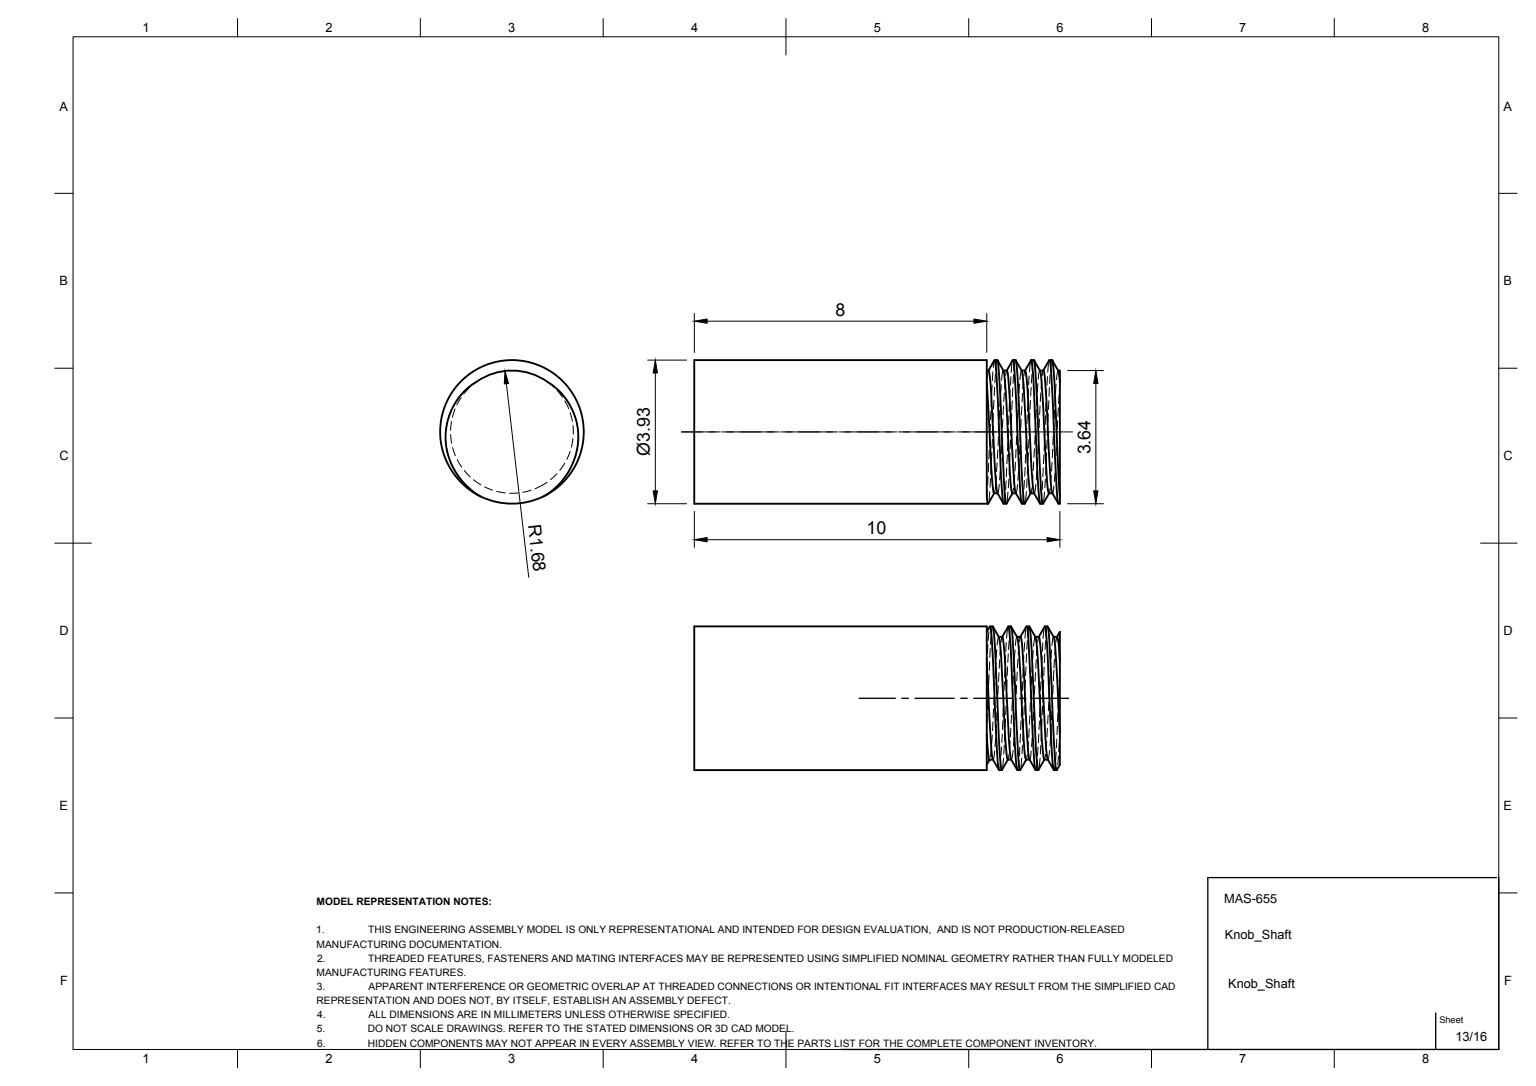
ISO-10303-21;
HEADER;
FILE_DESCRIPTION((''),'2;1');
FILE_NAME('Knob_Shaft.step','2026-10-09T11:34:15-07:00',(''),(''),'','','');
FILE_SCHEMA (('AUTOMOTIVE_DESIGN { 1 0 10303 214 3 1 1 }'));
ENDSEC;
DATA;
#10=MECHANICAL_DESIGN_GEOMETRIC_PRESENTATION_REPRESENTATION('',(#645),#117170);
#603=SHAPE_REPRESENTATION_RELATIONSHIP('SRR','None',#117258,#624) ;
#624=ADVANCED_BREP_SHAPE_REPRESENTATION('',(#666),#117166) ;
#645=STYLED_ITEM('',(#117355),#666) ;
#666=MANIFOLD_SOLID_BREP('Body1',#49074) ;
#761=FACE_BOUND('',#16411,.T.) ;
#1329=B_SPLINE_CURVE_WITH_KNOTS('',3,(#98755,#98756,#98757,#98758,#98759,
#98760,#98761,#98762,#98763,#98764,#98765,#98766,#98767,#98768,#98769,#98770,
#98771,#98772,#98773,#98774,#98775,#98776,#98777,#98778,#98779,#98780,#98781,
#98782,#98783,#98784,#98785,#98786,#98787,#98788,#98789,#98790,#98791,#98792,
#98793,#98794,#98795,#98796,#98797,#98798,#98799,#98800,#98801,#98802,#98803,
#98804,#98805,#98806,#98807,#98808,#98809,#98810,#98811,#98812,#98813,#98814,
#98815,#98816,#98817,#98818,#98819,#98820,#98821,#98822,#98823,#98824,#98825,
#98826,#98827,#98828,#98829,#98830,#98831,#98832,#98833,#98834),
 .UNSPECIFIED.,.F.,.F.,(4,2,2,2,2,2,2,2,2,2,2,2,2,2,2,2,2,2,2,2,2,2,2,2,
2,2,2,2,2,2,2,2,2,2,2,2,2,2,2,4),(-0.552597174673262,-0.552087978909823,
-0.543418802839412,-0.530986321926872,-0.515688074017889,-0.48901852632236,
-0.475795340291992,-0.469803806354904,-0.464827465085121,-0.456763485566357,
-0.446125790999932,-0.412222627640349,-0.396458552376544,-0.387367130961374,
-0.378547259036367,-0.364712615477276,-0.330180734182639,-0.312888098213682,
-0.306688567552087,-0.301731961915121,-0.294013236156573,-0.284057413245719,
-0.255750077060834,-0.235801635191627,-0.226007051069487,-0.217361674208648,
-0.205388809034252,-0.190982053575729,-0.163245460668606,-0.148987082829673,
-0.143002701370855,-0.137919038363949,-0.129466900901552,-0.118084610051148,
-0.0761832714464343,-0.0655381220499832,-0.0569431610964917,-0.0461350849955365,
-0.0209625497341524,-0.00261038353153479),.UNSPECIFIED.) ;
#1330=B_SPLINE_CURVE_WITH_KNOTS('',3,(#98837,#98838,#98839,#98840,#98841,
#98842,#98843,#98844,#98845,#98846,#98847,#98848,#98849,#98850,#98851,#98852,
#98853,#98854,#98855,#98856,#98857,#98858,#98859,#98860,#98861,#98862,#98863,
#98864,#98865,#98866,#98867,#98868,#98869,#98870,#98871,#98872,#98873,#98874,
#98875,#98876,#98877,#98878,#98879,#98880,#98881,#98882,#98883,#98884,#98885,
#98886),.UNSPECIFIED.,.F.,.F.,(4,2,2,2,2,2,2,2,2,2,2,2,2,2,2,2,2,2,2,2,
2,2,2,2,4),(-1.74405659608,-1.74024862573011,-1.7354490695973,-1.69761675650509,
-1.68391129329674,-1.67222759893424,-1.66298762114359,-1.6513941256668,
-1.6159137516185,-1.59065618245596,-1.58351862500578,-1.57860240737983,
-1.57213220939518,-1.537477246215,-1.51410228040979,-1.50437755876619,-1.49602419307963,
-1.48490892270242,-1.45580246644061,-1.43518707323026,-1.42657793655706,
-1.41966295247194,-1.41491213816115,-1.40875298679861,-1.40019423751868),
 .UNSPECIFIED.) ;
#1331=B_SPLINE_CURVE_WITH_KNOTS('',3,(#98891,#98892,#98893,#98894,#98895,
#98896,#98897,#98898,#98899,#98900,#98901,#98902,#98903,#98904,#98905,#98906,
#98907,#98908,#98909,#98910,#98911,#98912,#98913,#98914,#98915,#98916,#98917,
#98918,#98919,#98920,#98921,#98922,#98923,#98924,#98925,#98926,#98927,#98928,
#98929,#98930,#98931,#98932,#98933,#98934,#98935,#98936,#98937,#98938,#98939,
#98940,#98941,#98942,#98943,#98944,#98945,#98946,#98947,#98948,#98949,#98950,
#98951,#98952,#98953,#98954,#98955,#98956,#98957,#98958,#98959,#98960,#98961,
#98962,#98963,#98964,#98965,#98966,#98967,#98968,#98969,#98970,#98971,#98972,
#98973,#98974,#98975,#98976,#98977,#98978,#98979,#98980,#98981,#98982,#98983,
#98984,#98985,#98986,#98987,#98988,#98989,#98990,#98991,#98992,#98993,#98994,
#98995,#98996,#98997,#98998,#98999,#99000,#99001,#99002,#99003,#99004,#99005,
#99006,#99007,#99008,#99009,#99010,#99011,#99012,#99013,#99014,#99015,#99016,
#99017,#99018,#99019,#99020,#99021,#99022,#99023,#99024,#99025,#99026,#99027,
#99028,#99029,#99030,#99031,#99032),.UNSPECIFIED.,.F.,.F.,(4,2,2,2,2,2,
2,2,2,2,2,2,2,2,2,2,2,2,2,2,2,2,2,2,2,2,2,2,2,2,2,2,2,2,2,2,2,2,2,2,2,2,
2,2,2,2,2,2,2,2,2,2,2,2,2,2,2,2,2,2,2,2,2,2,2,2,2,2,2,2,4),(-1.60817871985196,
-1.60188697181691,-1.56617428509184,-1.54984087223545,-1.53688654692764,
-1.52815941900595,-1.51880035364366,-1.50119252756857,-1.46500106568252,
-1.45686511127176,-1.45016915517214,-1.4452730535428,-1.43827422610191,
-1.410720873795,-1.38068642007219,-1.37024130049903,-1.36171438017231,-1.35090239215872,
-1.31818186378263,-1.29333652168782,-1.28676822558853,-1.28186617089387,
-1.27471523608405,-1.25426210693583,-1.22954377855377,-1.21768281934354,
-1.20715919419871,-1.19863292932375,-1.18790517373592,-1.15426873354839,
-1.13057394980088,-1.12379973616585,-1.11890417570126,-1.11198677312076,
-1.08351739597117,-1.05355856892254,-1.04333843073385,-1.03479834540627,
-1.0238910563505,-0.996287106129177,-0.976227453852334,-0.964288354181759,
-0.958706935650863,-0.953530612564683,-0.944174280916242,-0.930866568317175,
-0.891101252113233,-0.880607430471217,-0.872083906506385,-0.861333132529412,
-0.836212201841313,-0.803368395572518,-0.796967637358088,-0.792061871113417,
-0.784846056910506,-0.775799271108273,-0.753119298036319,-0.728813193822705,
-0.717960451683399,-0.709427961265852,-0.69900655346212,-0.687320352856108,
-0.663461993928104,-0.641640554378349,-0.634492327931047,-0.62958458215972,
-0.622992165537731,-0.615037058215324,-0.580754809747541,-0.561631838713906,
-0.552597174673262),.UNSPECIFIED.) ;
#1332=B_SPLINE_CURVE_WITH_KNOTS('',3,(#99033,#99034,#99035,#99036,#99037,
#99038,#99039,#99040,#99041,#99042,#99043,#99044,#99045,#99046,#99047,#99048,
#99049,#99050,#99051,#99052,#99053,#99054,#99055,#99056,#99057,#99058,#99059,
#99060,#99061,#99062,#99063,#99064,#99065,#99066,#99067,#99068,#99069,#99070,
#99071,#99072,#99073,#99074,#99075,#99076,#99077,#99078,#99079,#99080,#99081,
#99082,#99083,#99084,#99085,#99086,#99087,#99088,#99089,#99090,#99091,#99092,
#99093,#99094,#99095,#99096,#99097,#99098,#99099,#99100,#99101,#99102,#99103,
#99104,#99105,#99106,#99107,#99108,#99109,#99110,#99111,#99112,#99113,#99114,
#99115,#99116,#99117,#99118,#99119,#99120,#99121,#99122,#99123,#99124,#99125,
#99126,#99127,#99128,#99129,#99130,#99131,#99132,#99133,#99134,#99135,#99136,
#99137,#99138,#99139,#99140,#99141,#99142,#99143,#99144,#99145,#99146,#99147,
#99148,#99149,#99150,#99151,#99152,#99153,#99154,#99155,#99156,#99157,#99158,
#99159,#99160,#99161,#99162,#99163,#99164,#99165,#99166,#99167,#99168,#99169,
#99170,#99171,#99172,#99173,#99174),.UNSPECIFIED.,.F.,.F.,(4,2,2,2,2,2,
2,2,2,2,2,2,2,2,2,2,2,2,2,2,2,2,2,2,2,2,2,2,2,2,2,2,2,2,2,2,2,2,2,2,2,2,
2,2,2,2,2,2,2,2,2,2,2,2,2,2,2,2,2,2,2,2,2,2,2,2,2,2,2,2,4),(-1.40019423751868,
-1.39059856461891,-1.35667598468847,-1.34290959713784,-1.33402342554946,
-1.32475733166678,-1.30815172066439,-1.27149851334997,-1.26331601166393,
-1.25658126033718,-1.25163113413534,-1.24446124954234,-1.22317299546722,
-1.19893660798004,-1.18715522406132,-1.17666499379619,-1.16809990650696,
-1.1572276585662,-1.12501053474387,-1.10009161766894,-1.09338700792244,
-1.08848701787225,-1.08148107106248,-1.05412084897453,-1.02341461347077,
-1.01315335487947,-1.00465968991157,-0.993932385879927,-0.961647123834745,
-0.936270329728169,-0.929746618015904,-0.92485572071812,-0.917705462014288,
-0.896911887819304,-0.872394270882754,-0.856049781705572,-0.846849723712218,
-0.838025885909813,-0.824390338136546,-0.790915249737361,-0.772823406769396,
-0.766455259867575,-0.761540972127907,-0.754256062725515,-0.745085604668567,
-0.721717226155916,-0.698227847610382,-0.687432671047302,-0.678903412564833,
-0.668436939858761,-0.637290397758027,-0.610963216220392,-0.603901842352647,
-0.599004302864263,-0.592366007013439,-0.56867953784493,-0.534621186939995,
-0.523939302554265,-0.515418012823645,-0.504864049701461,-0.492948449919942,
-0.467963543295212,-0.447868495117718,-0.440716118091854,-0.435815634952121,
-0.429254383948027,-0.40396129016647,-0.371801441673548,-0.360942278777566,
-0.35241374076114,-0.344414753026734),.UNSPECIFIED.) ;
#1333=B_SPLINE_CURVE_WITH_KNOTS('',3,(#99180,#99181,#99182,#99183,#99184,
#99185,#99186,#99187),.UNSPECIFIED.,.F.,.F.,(4,1,1,1,1,4),(21.9911559755827,
22.8773584072894,23.848998189505,24.8206379717207,25.7922777539364,26.2282473494963),
 .UNSPECIFIED.) ;
#1334=B_SPLINE_CURVE_WITH_KNOTS('',3,(#99188,#99189,#99190,#99191,#99192,
#99193,#99194,#99195,#99196,#99197,#99198,#99199,#99200,#99201,#99202,#99203,
#99204,#99205,#99206,#99207,#99208,#99209,#99210,#99211,#99212,#99213,#99214,
#99215,#99216,#99217,#99218,#99219,#99220,#99221,#99222,#99223,#99224,#99225,
#99226,#99227,#99228,#99229,#99230,#99231,#99232,#99233,#99234,#99235,#99236,
#99237),.UNSPECIFIED.,.F.,.F.,(4,2,2,2,2,2,2,2,2,2,2,2,2,2,2,2,2,2,2,2,
2,2,2,2,4),(-1.95186686044663,-1.9451727728085,-1.93967548024574,-1.93493962460603,
-1.92792572995927,-1.90152501587077,-1.87059969230919,-1.86007646778741,
-1.85155154543861,-1.84082680150995,-1.80717942800767,-1.78322121868641,
-1.77657104095611,-1.77167346878357,-1.76462252246752,-1.73795912356653,
-1.70712279558588,-1.69668728374485,-1.68816018090868,-1.67733734324366,
-1.64474656626435,-1.6204670242381,-1.61360536890348,-1.60871139946509,
-1.60817871985196),.UNSPECIFIED.) ;
#1335=B_SPLINE_CURVE_WITH_KNOTS('',3,(#99239,#99240,#99241,#99242,#99243,
#99244,#99245,#99246,#99247,#99248,#99249,#99250,#99251,#99252,#99253,#99254,
#99255,#99256,#99257,#99258,#99259,#99260,#99261,#99262,#99263,#99264,#99265,
#99266,#99267,#99268,#99269,#99270,#99271,#99272,#99273,#99274,#99275,#99276,
#99277,#99278,#99279,#99280,#99281,#99282,#99283,#99284,#99285,#99286,#99287,
#99288),.UNSPECIFIED.,.F.,.F.,(4,2,2,2,2,2,2,2,2,2,2,2,2,2,2,2,2,2,2,2,
2,2,2,2,4),(-0.344414753026734,-0.342008927015211,-0.330348848139387,-0.306608071890107,
-0.284590171653946,-0.277445774946498,-0.272544248501529,-0.265971783203178,
-0.240098440585068,-0.20869911101062,-0.197899738456524,-0.189367850672706,
-0.179070471921566,-0.14943964187475,-0.120798932996502,-0.113894953777187,
-0.109001470737898,-0.102221682855731,-0.0939417781600824,-0.0750956593381936,
-0.0453269004351953,-0.0345663159816099,-0.0260362888104047,-0.0179340362145887,
-0.000450587274275642),.UNSPECIFIED.) ;
#1336=B_SPLINE_CURVE_WITH_KNOTS('',3,(#99289,#99290,#99291,#99292,#99293,
#99294,#99295,#99296,#99297),.UNSPECIFIED.,.F.,.F.,(4,1,1,1,1,1,4),(21.991153076628,
22.3032518321271,23.2748916143428,24.2465313965585,25.2181711787741,26.1898109609898,
26.2282235152758),.UNSPECIFIED.) ;
#1337=B_SPLINE_CURVE_WITH_KNOTS('',3,(#99303,#99304,#99305,#99306,#99307,
#99308,#99309,#99310,#99311,#99312,#99313,#99314,#99315,#99316,#99317,#99318,
#99319,#99320,#99321,#99322,#99323,#99324,#99325,#99326,#99327,#99328,#99329,
#99330,#99331,#99332,#99333,#99334,#99335,#99336,#99337,#99338,#99339,#99340,
#99341,#99342,#99343,#99344,#99345,#99346,#99347,#99348,#99349,#99350,#99351,
#99352,#99353,#99354,#99355,#99356,#99357,#99358,#99359,#99360,#99361,#99362,
#99363,#99364,#99365,#99366,#99367,#99368,#99369,#99370,#99371,#99372,#99373,
#99374,#99375,#99376,#99377,#99378,#99379,#99380,#99381,#99382,#99383,#99384,
#99385,#99386,#99387,#99388,#99389,#99390,#99391,#99392,#99393,#99394,#99395,
#99396,#99397,#99398,#99399,#99400,#99401,#99402,#99403,#99404,#99405,#99406,
#99407,#99408,#99409,#99410,#99411,#99412,#99413,#99414,#99415,#99416,#99417,
#99418,#99419,#99420),.UNSPECIFIED.,.F.,.F.,(4,3,3,3,3,3,3,3,3,3,3,3,3,
3,3,3,3,3,3,3,3,3,3,3,3,3,3,3,3,3,3,3,3,3,3,3,3,3,3,4),(28.2743338823083,
28.3918577143769,28.5096434298568,28.627852053642,28.7071971005834,28.8171687317807,
28.9269585285024,29.0366468598356,29.1462735902616,29.2558784995052,29.3655762062641,
29.4753180348027,29.5852552742705,29.6788368827991,29.788799074535,29.8985797766649,
30.0082592302568,30.1178773128371,30.2274738174318,30.337163559117,30.4468976537998,
30.5568276341267,30.6504766650147,30.7603622112468,30.8700658671167,30.9796680949326,
31.0892089139856,31.1987282589466,31.3083416196759,31.4179996566885,31.5278550625658,
31.6221164472304,31.7332153421388,31.8431388376641,31.9529583560026,32.0627135252056,
32.1747620455285,32.2845571568611,32.3977323816792,32.5109076064973),
 .UNSPECIFIED.) ;
#1338=B_SPLINE_CURVE_WITH_KNOTS('',3,(#99421,#99422,#99423,#99424,#99425,
#99426),.UNSPECIFIED.,.F.,.F.,(4,1,1,4),(26.2282473494963,26.763917536152,
27.7355573183677,28.2743338823083),.UNSPECIFIED.) ;
#1339=B_SPLINE_CURVE_WITH_KNOTS('',3,(#99428,#99429,#99430,#99431,#99432,
#99433),.UNSPECIFIED.,.F.,.F.,(4,1,1,4),(26.2282235152758,27.1614507432055,
28.1330905254212,28.2743338823083),.UNSPECIFIED.) ;
#1340=B_SPLINE_CURVE_WITH_KNOTS('',3,(#99434,#99435,#99436,#99437,#99438,
#99439,#99440,#99441,#99442,#99443,#99444,#99445,#99446,#99447,#99448,#99449,
#99450,#99451,#99452,#99453,#99454,#99455,#99456,#99457,#99458,#99459,#99460,
#99461,#99462,#99463,#99464,#99465,#99466,#99467,#99468,#99469,#99470,#99471,
#99472,#99473,#99474,#99475,#99476,#99477,#99478,#99479,#99480,#99481,#99482,
#99483,#99484,#99485,#99486,#99487,#99488,#99489,#99490,#99491,#99492,#99493,
#99494,#99495,#99496,#99497,#99498,#99499,#99500,#99501,#99502,#99503,#99504,
#99505,#99506,#99507,#99508,#99509,#99510,#99511,#99512,#99513,#99514,#99515,
#99516,#99517,#99518,#99519,#99520,#99521,#99522,#99523,#99524,#99525,#99526,
#99527,#99528,#99529,#99530,#99531,#99532,#99533),.UNSPECIFIED.,.F.,.F.,
(4,2,2,2,2,2,2,2,2,2,2,2,2,2,2,2,2,2,2,2,2,2,2,2,2,2,2,2,2,2,2,2,2,2,2,
2,2,2,2,2,2,2,2,2,2,2,2,2,2,4),(0.71239184097541,0.712394397109961,0.721192745130405,
0.734671500759373,0.752082681774165,0.785389301747164,0.792361482669575,
0.797255532613846,0.803969694657684,0.812137997382168,0.848691796614872,
0.866018595123892,0.875338577534295,0.884075623393995,0.897136442047152,
0.913687074888232,0.949536070553263,0.956049447834536,0.960945375490526,
0.968005360973277,0.976776672286265,0.997997587656753,1.02408233804888,
1.03492929727984,1.04346381630968,1.05372425154729,1.08322460952202,1.11212627116881,
1.11900052456233,1.12389412033395,1.13070424102562,1.13903754049952,1.1581264104363,
1.18716937335988,1.19807583912576,1.20661269099351,1.21682479433147,1.24642058771588,
1.27539968756184,1.28226660540231,1.28715951003292,1.293974316854,1.30231588418635,
1.3214434868297,1.35042743331143,1.36133490544489,1.36987153696253,1.38008212757361,
1.40961316219556,1.42438117464762),.UNSPECIFIED.) ;
#1341=B_SPLINE_CURVE_WITH_KNOTS('',3,(#99539,#99540,#99541,#99542,#99543,
#99544,#99545,#99546),.UNSPECIFIED.,.F.,.F.,(4,1,1,1,1,4),(-27.2059139020388,
-26.2342741198231,-25.2626343376075,-24.2909945553918,-23.3193547731761,
-22.9423101986588),.UNSPECIFIED.) ;
#1342=B_SPLINE_CURVE_WITH_KNOTS('',3,(#99548,#99549,#99550,#99551,#99552,
#99553,#99554,#99555,#99556,#99557,#99558,#99559,#99560,#99561,#99562,#99563,
#99564,#99565,#99566,#99567,#99568,#99569,#99570,#99571,#99572,#99573,#99574,
#99575,#99576,#99577,#99578,#99579,#99580,#99581,#99582,#99583,#99584,#99585,
#99586,#99587,#99588,#99589,#99590,#99591,#99592,#99593,#99594,#99595,#99596,
#99597,#99598,#99599,#99600,#99601,#99602,#99603,#99604,#99605,#99606,#99607,
#99608,#99609,#99610,#99611,#99612,#99613,#99614,#99615,#99616,#99617,#99618,
#99619,#99620,#99621,#99622,#99623,#99624,#99625,#99626,#99627,#99628,#99629,
#99630,#99631,#99632,#99633,#99634,#99635,#99636,#99637,#99638,#99639,#99640,
#99641,#99642,#99643,#99644,#99645,#99646,#99647,#99648,#99649,#99650,#99651,
#99652,#99653,#99654,#99655,#99656,#99657,#99658,#99659,#99660,#99661,#99662,
#99663,#99664,#99665,#99666,#99667,#99668,#99669,#99670,#99671,#99672,#99673,
#99674,#99675,#99676,#99677,#99678,#99679,#99680,#99681,#99682,#99683,#99684,
#99685,#99686,#99687,#99688,#99689,#99690,#99691,#99692,#99693,#99694,#99695,
#99696,#99697,#99698,#99699,#99700,#99701,#99702,#99703,#99704,#99705,#99706,
#99707,#99708,#99709,#99710,#99711,#99712,#99713,#99714,#99715,#99716,#99717,
#99718,#99719,#99720,#99721,#99722,#99723,#99724,#99725,#99726,#99727,#99728,
#99729,#99730,#99731,#99732,#99733,#99734,#99735,#99736,#99737,#99738,#99739,
#99740),.UNSPECIFIED.,.F.,.F.,(4,3,3,3,3,3,3,3,3,3,3,3,3,3,3,3,3,3,3,3,
3,3,3,3,3,3,3,3,3,3,3,3,3,3,3,3,3,3,3,3,3,3,3,3,3,3,3,3,3,3,3,3,3,3,3,3,
3,3,3,3,3,3,3,3,4),(-22.9423049617328,-22.8359148801892,-22.7294989965987,
-22.6229467860948,-22.5163206965427,-22.4094948198208,-22.3477149909605,
-22.2419915581329,-22.1337520144594,-22.0282967847123,-21.9229011330953,
-21.8175296898858,-21.7071660696005,-21.601672616691,-21.496111283468,-21.3903880127637,
-21.3760752087448,-21.2703449398838,-21.1621062507144,-21.0566433996443,
-20.9512398559663,-20.8458602624753,-20.7355040534888,-20.6300018920914,
-20.5244316643326,-20.4186992962299,-20.4044354265291,-20.2987232478075,
-20.1904822973707,-20.0850383870169,-19.9796540446497,-19.8742938798852,
-19.7639193209922,-19.6584369302253,-19.5528865727019,-19.4471740767142,
-19.4327956443134,-19.3270755254136,-19.2188355674991,-19.1133834622704,
-19.0079908543491,-18.9026223676423,-18.7922557412562,-18.6867649852429,
-18.5812062554424,-18.4754854358354,-18.4611558620978,-18.3554360769796,
-18.2471960773424,-18.1417442640643,-18.0363519316643,-17.9309837035316,
-17.8206167976192,-17.7151262543179,-17.6095677211043,-17.5038470738284,
-17.4895160798821,-17.385308618441,-17.2812327055803,-17.1772506824177,
-17.0733250178827,-16.9693644269059,-16.8653930128412,-16.7612777927426,
-16.6591196549159),.UNSPECIFIED.) ;
#1343=B_SPLINE_CURVE_WITH_KNOTS('',3,(#99742,#99743,#99744,#99745,#99746,
#99747,#99748,#99749,#99750,#99751,#99752,#99753,#99754,#99755,#99756,#99757,
#99758,#99759,#99760,#99761,#99762,#99763,#99764,#99765,#99766,#99767,#99768,
#99769,#99770,#99771,#99772,#99773,#99774,#99775,#99776,#99777,#99778,#99779,
#99780,#99781,#99782,#99783,#99784,#99785,#99786,#99787,#99788,#99789,#99790,
#99791,#99792,#99793,#99794,#99795,#99796,#99797,#99798,#99799,#99800,#99801,
#99802,#99803,#99804,#99805,#99806,#99807,#99808,#99809,#99810,#99811,#99812,
#99813,#99814,#99815,#99816,#99817,#99818,#99819,#99820,#99821,#99822,#99823,
#99824,#99825,#99826,#99827,#99828,#99829,#99830,#99831,#99832,#99833,#99834,
#99835,#99836,#99837,#99838,#99839,#99840,#99841,#99842,#99843,#99844,#99845,
#99846,#99847,#99848,#99849,#99850,#99851,#99852,#99853,#99854,#99855,#99856,
#99857,#99858,#99859,#99860,#99861,#99862,#99863,#99864,#99865,#99866,#99867,
#99868,#99869,#99870,#99871,#99872,#99873,#99874,#99875,#99876,#99877,#99878,
#99879,#99880,#99881,#99882,#99883,#99884,#99885,#99886,#99887,#99888,#99889,
#99890,#99891,#99892,#99893,#99894,#99895,#99896,#99897,#99898,#99899,#99900,
#99901,#99902,#99903,#99904,#99905,#99906,#99907,#99908,#99909,#99910,#99911,
#99912,#99913,#99914,#99915,#99916,#99917,#99918,#99919,#99920,#99921,#99922,
#99923,#99924,#99925,#99926,#99927,#99928,#99929,#99930,#99931,#99932,#99933,
#99934),.UNSPECIFIED.,.F.,.F.,(4,3,3,3,3,3,3,3,3,3,3,3,3,3,3,3,3,3,3,3,
3,3,3,3,3,3,3,3,3,3,3,3,3,3,3,3,3,3,3,3,3,3,3,3,3,3,3,3,3,3,3,3,3,3,3,3,
3,3,3,3,3,3,3,3,4),(-16.6591196545535,-16.5178762976664,-16.4121571798967,
-16.303917096841,-16.1984659957846,-16.0930743902226,-15.9877069023141,
-15.8773393055983,-15.7718495275461,-15.6662917675439,-15.5605718993772,
-15.5462365154507,-15.4405175111645,-15.3322774139233,-15.2268264264059,
-15.1214349340659,-15.0160675588606,-14.9056998524542,-14.8002101844403,
-14.6946525334436,-14.5889327720487,-14.5745967332351,-14.4688778257925,
-14.3606377164459,-14.2551868319594,-14.1497954446504,-14.0444281762974,
-13.9340603699779,-13.8285708121443,-13.7230132723779,-13.6172936229251,
-13.6029569510194,-13.497238049513,-13.3889979394243,-13.283547057409,-13.1781556712829,
-13.0727884028267,-12.9624205943209,-12.8569310331724,-12.7513734889853,
-12.6456538335856,-12.6313171688037,-12.5255981556417,-12.41735805951,-12.3119070682978,
-12.2065155741889,-12.1011481991378,-11.9907804960004,-11.8852908329427,
-11.7797331885556,-11.6740134360523,-11.6596773865881,-11.5539582669364,
-11.4457181841159,-11.340267082276,-11.2348754763391,-11.1295079884633,
-11.0191403924406,-10.9136506154393,-10.8080928568386,-10.7023729905574,
-10.6880376043724,-10.5637109947364,-10.440558501415,-10.3759343476562),
 .UNSPECIFIED.) ;
#1344=B_SPLINE_CURVE_WITH_KNOTS('',3,(#99936,#99937,#99938,#99939,#99940,
#99941,#99942,#99943,#99944,#99945,#99946,#99947,#99948,#99949,#99950,#99951,
#99952,#99953,#99954,#99955,#99956,#99957,#99958,#99959,#99960,#99961,#99962,
#99963,#99964,#99965,#99966,#99967,#99968,#99969,#99970,#99971,#99972,#99973,
#99974,#99975,#99976,#99977,#99978,#99979,#99980,#99981,#99982,#99983,#99984,
#99985,#99986,#99987,#99988,#99989,#99990,#99991,#99992,#99993,#99994,#99995,
#99996,#99997,#99998,#99999,#100000,#100001,#100002,#100003,#100004,#100005,
#100006,#100007,#100008,#100009,#100010,#100011,#100012,#100013,#100014,
#100015,#100016,#100017,#100018,#100019,#100020,#100021,#100022,#100023,
#100024,#100025,#100026,#100027,#100028,#100029,#100030,#100031,#100032,
#100033,#100034,#100035,#100036,#100037,#100038,#100039,#100040,#100041,
#100042,#100043,#100044,#100045,#100046,#100047,#100048,#100049,#100050,
#100051,#100052,#100053,#100054,#100055,#100056,#100057,#100058,#100059,
#100060,#100061,#100062,#100063,#100064,#100065,#100066,#100067,#100068,
#100069,#100070,#100071,#100072,#100073,#100074,#100075,#100076,#100077,
#100078,#100079,#100080,#100081,#100082,#100083,#100084,#100085,#100086,
#100087,#100088,#100089,#100090,#100091,#100092,#100093,#100094,#100095,
#100096,#100097,#100098,#100099,#100100,#100101,#100102,#100103,#100104,
#100105,#100106,#100107,#100108,#100109,#100110,#100111,#100112,#100113,
#100114,#100115,#100116,#100117,#100118,#100119,#100120,#100121,#100122,
#100123,#100124,#100125,#100126,#100127,#100128,#100129,#100130,#100131),
 .UNSPECIFIED.,.F.,.F.,(4,3,3,3,3,3,3,3,3,3,3,3,3,3,3,3,3,3,3,3,3,3,3,3,
3,3,3,3,3,3,3,3,3,3,3,3,3,3,3,3,3,3,3,3,3,3,3,3,3,3,3,3,3,3,3,3,3,3,3,3,
3,3,3,3,3,4),(-10.3759343473739,-10.2708182319272,-10.1657261816089,-10.0606224885171,
-9.95540605732621,-9.85012227155168,-9.7446668862292,-9.71639782215672,
-9.61067792538572,-9.50243793970514,-9.39698607994724,-9.291593725295,-9.18622549910132,
-9.07585863431126,-8.97036815335541,-8.86480970328484,-8.75908916785834,
-8.74475803994105,-8.6390379713579,-8.53079800715383,-8.42534592287132,
-8.31995332497796,-8.21458483739726,-8.10421819247929,-7.99872740836975,
-7.89316864110053,-7.7874477710884,-7.77311825772537,-7.66740649115993,
-7.55916548920365,-7.45372175043135,-7.348337490219,-7.24297731831515,-7.13260260761379,
-7.02711998672144,-6.92156932230534,-6.81585641345591,-6.8014784755097,
-6.6957468880536,-6.58750836370865,-6.48204496374827,-6.37664115733222,
-6.27126158683108,-6.16090586344681,-6.05540443841166,-5.9498351926574,
-5.84410414555403,-5.82983869329403,-5.72411618037325,-5.61587652171139,
-5.51042167490583,-5.40502620661422,-5.29965474740967,-5.18929078832684,
-5.08379682173855,-4.9782348034796,-4.87251061123387,-4.85819891107836,
-4.75396836036899,-4.64987198240714,-4.54587213384773,-4.44193130364946,
-4.33797515998441,-4.23400960594329,-4.12994645754084,-4.09274904045272),
 .UNSPECIFIED.) ;
#1345=B_SPLINE_CURVE_WITH_KNOTS('',3,(#100133,#100134,#100135,#100136,#100137,
#100138,#100139,#100140,#100141,#100142,#100143,#100144,#100145,#100146,
#100147,#100148,#100149,#100150,#100151,#100152,#100153,#100154,#100155,
#100156,#100157,#100158,#100159,#100160,#100161,#100162,#100163,#100164,
#100165,#100166,#100167,#100168,#100169,#100170,#100171,#100172,#100173,
#100174,#100175,#100176,#100177,#100178,#100179,#100180,#100181,#100182,
#100183,#100184,#100185,#100186,#100187,#100188,#100189,#100190,#100191,
#100192,#100193),.UNSPECIFIED.,.F.,.F.,(4,3,3,3,3,3,3,3,3,3,3,3,3,3,3,3,
3,3,3,3,4),(-4.09274904019418,-3.94994229097354,-3.88655912886269,-3.7806981588848,
-3.67247580735508,-3.56688347781595,-3.46135127622131,-3.35584405875722,
-3.24561288072967,-3.13998714819308,-3.03429486644919,-2.92844341909598,
-2.91491934664702,-2.80976849252938,-2.7057785484878,-2.60187950128122,
-2.49803373370174,-2.39195342870279,-2.28805068804784,-2.18088160087689,
-2.07371251370594),.UNSPECIFIED.) ;
#1346=B_SPLINE_CURVE_WITH_KNOTS('',3,(#100197,#100198,#100199,#100200,#100201),
 .UNSPECIFIED.,.F.,.F.,(4,1,4),(0.,0.971639782215675,1.12201628671505),
 .UNSPECIFIED.) ;
#1347=B_SPLINE_CURVE_WITH_KNOTS('',3,(#100203,#100204,#100205,#100206,#100207,
#100208,#100209,#100210,#100211,#100212,#100213,#100214,#100215,#100216,
#100217,#100218,#100219,#100220,#100221,#100222,#100223,#100224,#100225,
#100226,#100227,#100228,#100229,#100230,#100231,#100232,#100233,#100234,
#100235,#100236,#100237,#100238,#100239,#100240,#100241,#100242,#100243,
#100244,#100245,#100246,#100247,#100248,#100249,#100250,#100251,#100252,
#100253,#100254,#100255,#100256,#100257,#100258,#100259,#100260,#100261,
#100262,#100263,#100264,#100265,#100266,#100267,#100268,#100269,#100270,
#100271,#100272,#100273,#100274,#100275,#100276,#100277,#100278,#100279,
#100280,#100281,#100282,#100283,#100284,#100285,#100286,#100287,#100288,
#100289,#100290,#100291,#100292,#100293,#100294,#100295,#100296,#100297,
#100298,#100299,#100300,#100301,#100302,#100303,#100304,#100305,#100306,
#100307,#100308,#100309,#100310,#100311,#100312,#100313,#100314,#100315,
#100316,#100317,#100318,#100319,#100320,#100321,#100322,#100323,#100324,
#100325,#100326,#100327,#100328,#100329,#100330,#100331,#100332,#100333,
#100334,#100335,#100336,#100337,#100338,#100339,#100340,#100341,#100342,
#100343,#100344,#100345,#100346,#100347,#100348,#100349,#100350,#100351,
#100352,#100353,#100354,#100355,#100356,#100357,#100358,#100359,#100360,
#100361,#100362,#100363,#100364,#100365,#100366,#100367,#100368,#100369,
#100370,#100371,#100372,#100373,#100374,#100375,#100376,#100377,#100378,
#100379,#100380,#100381,#100382,#100383,#100384,#100385,#100386,#100387,
#100388,#100389,#100390,#100391,#100392,#100393,#100394,#100395),
 .UNSPECIFIED.,.F.,.F.,(4,3,3,3,3,3,3,3,3,3,3,3,3,3,3,3,3,3,3,3,3,3,3,3,
3,3,3,3,3,3,3,3,3,3,3,3,3,3,3,3,3,3,3,3,3,3,3,3,3,3,3,3,3,3,3,3,3,3,3,3,
3,3,3,3,4),(1.12201628671505,1.22572984062012,1.3293396932848,1.43288383968884,
1.53640017806041,1.63999591211869,1.74362768694738,1.84744171560355,1.94327956443135,
2.04897598618115,2.15721890623938,2.2626389507752,2.3679965240157,2.4733270907322,
2.58372515471091,2.68917132531124,2.79468322907709,2.900354428491,2.91491934664702,
3.02076970287158,3.12899338112047,3.2345812937059,3.34011138403074,3.44561879250706,
3.55585387659597,3.66148554028109,3.76718573243698,3.87304781693433,3.8865591288627,
3.99221130516841,4.10045975590715,4.20584169368149,4.31116350983744,4.41646070071832,
4.52689525330833,4.6323142796995,4.73780119575579,4.84345058285624,4.85819891107837,
4.96392234279262,5.0721618866053,5.17761711523643,5.28301276573926,5.38838420783775,
5.49874782920182,5.60424128101974,5.70980261315803,5.81552588279539,5.82983869329404,
5.93556896205594,6.04380765123766,6.14927050221238,6.25467404579622,6.36005363919464,
6.47040984827341,6.57591200958229,6.68148223725401,6.78721460527208,6.80147847550972,
6.90810448169561,7.01457253381657,7.12090167820117,7.22714842106499,7.33336029947649,
7.40520159389472),.UNSPECIFIED.) ;
#1348=B_SPLINE_CURVE_WITH_KNOTS('',3,(#100397,#100398,#100399,#100400,#100401,
#100402,#100403,#100404,#100405,#100406,#100407,#100408,#100409,#100410,
#100411,#100412,#100413,#100414,#100415,#100416,#100417,#100418,#100419,
#100420,#100421,#100422,#100423,#100424,#100425,#100426,#100427,#100428,
#100429,#100430,#100431,#100432,#100433,#100434,#100435,#100436,#100437,
#100438,#100439,#100440,#100441,#100442,#100443,#100444,#100445,#100446,
#100447,#100448,#100449,#100450,#100451,#100452,#100453,#100454,#100455,
#100456,#100457,#100458,#100459,#100460,#100461,#100462,#100463,#100464,
#100465,#100466,#100467,#100468,#100469,#100470,#100471,#100472,#100473,
#100474,#100475,#100476,#100477,#100478,#100479,#100480,#100481,#100482,
#100483,#100484,#100485,#100486,#100487,#100488,#100489,#100490,#100491,
#100492,#100493,#100494,#100495,#100496,#100497,#100498,#100499,#100500,
#100501,#100502,#100503,#100504,#100505,#100506,#100507,#100508,#100509,
#100510,#100511,#100512,#100513,#100514,#100515,#100516,#100517,#100518,
#100519,#100520,#100521,#100522,#100523,#100524,#100525,#100526,#100527,
#100528,#100529,#100530,#100531,#100532,#100533,#100534,#100535,#100536,
#100537,#100538,#100539,#100540,#100541,#100542,#100543,#100544,#100545,
#100546,#100547,#100548,#100549,#100550,#100551,#100552,#100553,#100554,
#100555,#100556,#100557,#100558,#100559,#100560,#100561,#100562,#100563,
#100564,#100565,#100566,#100567,#100568,#100569,#100570,#100571,#100572,
#100573,#100574,#100575,#100576,#100577,#100578,#100579,#100580,#100581,
#100582,#100583,#100584,#100585,#100586,#100587,#100588,#100589,#100590,
#100591,#100592),.UNSPECIFIED.,.F.,.F.,(4,3,3,3,3,3,3,3,3,3,3,3,3,3,3,3,
3,3,3,3,3,3,3,3,3,3,3,3,3,3,3,3,3,3,3,3,3,3,3,3,3,3,3,3,3,3,3,3,3,3,3,3,
3,3,3,3,3,3,3,3,3,3,3,3,3,4),(7.40520159423053,7.52274823355723,7.64076675914912,
7.75933359401983,7.77311825772539,7.87883837651618,7.98707833444429,8.09253043956017,
8.1979230473676,8.30329153395943,8.41365816045484,8.51914891635246,8.624707646037,
8.73042846552869,8.74475803994107,8.85047782504704,8.95871782468575,9.06416963794981,
9.16956197033504,9.27493019845273,9.38529710437873,9.49078764766358,9.59634618086029,
9.70206682811849,9.71639782215674,9.8221160929373,9.93035628186669,10.0358065051139,
10.1411972239824,10.2465638178459,10.3569322644775,10.4624211405789,10.5679779967512,
10.6736969647547,10.6880376043724,10.7937567221263,10.901996805184,11.0074479062241,
11.1128395117695,11.2182069996615,11.3285745963931,11.4340643744287,11.5396221344144,
11.6453420025645,11.6596773865881,11.7653963908742,11.8736364881154,11.9790874756325,
12.0844789679723,12.1898463431774,12.300214049584,12.4057037175975,12.5112613685939,
12.6169811299884,12.6313171688038,12.7370360762483,12.8452761855947,12.9507270700831,
13.0561184573942,13.1614857257493,13.2718535320668,13.3773430899027,13.4829006296713,
13.5886202791265,13.6029569510194,13.6883869010744),.UNSPECIFIED.) ;
#1349=B_SPLINE_CURVE_WITH_KNOTS('',3,(#100594,#100595,#100596,#100597,#100598,
#100599,#100600,#100601,#100602,#100603,#100604,#100605,#100606,#100607,
#100608,#100609,#100610,#100611,#100612,#100613,#100614,#100615,#100616,
#100617,#100618,#100619,#100620,#100621,#100622,#100623,#100624,#100625,
#100626,#100627,#100628,#100629,#100630,#100631,#100632,#100633,#100634,
#100635,#100636,#100637,#100638,#100639,#100640,#100641,#100642,#100643,
#100644,#100645,#100646,#100647,#100648,#100649,#100650,#100651,#100652,
#100653,#100654,#100655,#100656,#100657,#100658,#100659,#100660,#100661,
#100662,#100663,#100664,#100665,#100666,#100667,#100668,#100669,#100670,
#100671,#100672,#100673,#100674,#100675,#100676,#100677,#100678,#100679,
#100680,#100681,#100682,#100683,#100684,#100685,#100686,#100687,#100688,
#100689,#100690,#100691,#100692,#100693,#100694,#100695,#100696,#100697,
#100698,#100699,#100700,#100701,#100702,#100703,#100704,#100705,#100706,
#100707,#100708,#100709,#100710,#100711,#100712,#100713,#100714,#100715,
#100716,#100717,#100718,#100719,#100720,#100721,#100722,#100723,#100724,
#100725,#100726,#100727,#100728,#100729,#100730,#100731,#100732,#100733,
#100734,#100735,#100736,#100737,#100738,#100739,#100740,#100741,#100742,
#100743,#100744,#100745,#100746,#100747,#100748,#100749,#100750,#100751,
#100752,#100753,#100754,#100755,#100756,#100757,#100758,#100759,#100760,
#100761,#100762,#100763,#100764,#100765,#100766,#100767,#100768,#100769,
#100770,#100771,#100772,#100773,#100774,#100775,#100776,#100777,#100778,
#100779,#100780,#100781,#100782,#100783,#100784,#100785,#100786),
 .UNSPECIFIED.,.F.,.F.,(4,3,3,3,3,3,3,3,3,3,3,3,3,3,3,3,3,3,3,3,3,3,3,3,
3,3,3,3,3,3,3,3,3,3,3,3,3,3,3,3,3,3,3,3,3,3,3,3,3,3,3,3,3,3,3,3,3,3,3,3,
3,3,3,3,4),(13.6883869014632,13.7928966428815,13.8972545308479,14.001529543701,
14.1057588206298,14.2099794369136,14.314293022429,14.4186584614246,14.5231928822222,
14.5745967332351,14.6803157463967,14.7885558425284,14.8940068337404,14.9993983278492,
15.1047657029,15.2151334060377,15.3206230690952,15.4261807134823,15.5319004659856,
15.5462365154508,15.6519556350861,15.7601957179086,15.865646819732,15.9710384256524,
16.0764059135115,16.1867735095503,16.2922632865352,16.3978210451198,16.5035409113853,
16.5178762976665,16.6235945194864,16.7318347145359,16.8372849174012,16.9426756265115,
17.0480422212251,17.1584106858893,17.2638995893294,17.3694564819601,17.4751754990101,
17.4895160798821,17.5952359766356,17.7034759623184,17.8089278220601,17.9143201766965,
18.019688402875,18.1300552676807,18.2355457486229,18.3411041986802,18.4468247340942,
18.4611558620978,18.5668759305656,18.6751158947841,18.7805679789512,18.8859605767293,
18.9913290641955,19.101695709225,19.2071864932224,19.3127452603802,19.4184661302833,
19.4327956443135,19.5414241997911,19.6498165890499,19.7580693322231,19.8661877984924,
19.9715722082541),.UNSPECIFIED.) ;
#1350=B_SPLINE_CURVE_WITH_KNOTS('',3,(#100788,#100789,#100790,#100791,#100792,
#100793,#100794,#100795,#100796,#100797,#100798,#100799,#100800,#100801,
#100802,#100803,#100804,#100805,#100806,#100807,#100808,#100809,#100810,
#100811,#100812,#100813,#100814,#100815,#100816,#100817,#100818,#100819,
#100820,#100821,#100822,#100823,#100824,#100825,#100826,#100827,#100828,
#100829,#100830,#100831,#100832,#100833,#100834,#100835,#100836,#100837,
#100838,#100839,#100840,#100841,#100842,#100843,#100844,#100845,#100846,
#100847,#100848,#100849,#100850,#100851,#100852,#100853,#100854,#100855,
#100856,#100857,#100858,#100859,#100860,#100861,#100862,#100863,#100864,
#100865,#100866,#100867,#100868,#100869,#100870,#100871,#100872,#100873,
#100874,#100875,#100876,#100877,#100878,#100879,#100880,#100881,#100882,
#100883,#100884,#100885,#100886,#100887,#100888,#100889,#100890,#100891,
#100892,#100893,#100894,#100895,#100896,#100897,#100898,#100899,#100900,
#100901,#100902,#100903,#100904,#100905,#100906,#100907,#100908,#100909,
#100910,#100911,#100912,#100913,#100914,#100915,#100916,#100917,#100918,
#100919,#100920,#100921,#100922,#100923,#100924,#100925,#100926,#100927,
#100928,#100929,#100930,#100931,#100932,#100933,#100934,#100935,#100936,
#100937,#100938,#100939,#100940,#100941,#100942,#100943,#100944),
 .UNSPECIFIED.,.F.,.F.,(4,3,3,3,3,3,3,3,3,3,3,3,3,3,3,3,3,3,3,3,3,3,3,3,
3,3,3,3,3,3,3,3,3,3,3,3,3,3,3,3,3,3,3,3,3,3,3,3,3,3,3,3,4),(19.971572208661,
20.0845648157855,20.1977995689991,20.3114399446563,20.4044354265292,20.510167013901,
20.6184055382565,20.7238689381274,20.8292727444523,20.9346523148608,21.0450080383318,
21.1505094632704,21.2560787089269,21.361809755931,21.3760752087448,21.4817977206012,
21.5900373793961,21.6954922251061,21.8008876922933,21.9062591503856,22.0166231105293,
22.1221170759983,22.2276790931361,22.3334032842653,22.3477149909605,22.4533638124416,
22.5616126825334,22.666993223323,22.7723143699649,22.8776116177223,22.9880474065858,
23.0934683050467,23.1989577176671,23.304610464124,23.3193547731762,23.4252157407445,
23.5334380925754,23.6390304199759,23.7445626195405,23.850069835088,23.9603010151639,
24.0659267460978,24.1716190263506,24.2774704723827,24.2909945553918,24.3962128895577,
24.5002027571533,24.6041017693643,24.7079475432931,24.8141459646495,24.9180489703703,
25.0253950995445,25.1327412287187),.UNSPECIFIED.) ;
#1351=B_SPLINE_CURVE_WITH_KNOTS('',3,(#100945,#100946,#100947,#100948),
 .UNSPECIFIED.,.F.,.F.,(4,4),(-0.0366228796273741,0.),.UNSPECIFIED.) ;
#1352=B_SPLINE_CURVE_WITH_KNOTS('',3,(#100953,#100954,#100955,#100956,#100957,
#100958,#100959,#100960,#100961,#100962,#100963,#100964,#100965,#100966,
#100967,#100968,#100969,#100970,#100971,#100972,#100973,#100974,#100975,
#100976,#100977,#100978,#100979,#100980,#100981,#100982,#100983,#100984,
#100985,#100986,#100987,#100988,#100989,#100990,#100991,#100992,#100993,
#100994,#100995,#100996,#100997,#100998,#100999,#101000,#101001,#101002,
#101003,#101004,#101005,#101006,#101007,#101008,#101009,#101010,#101011,
#101012,#101013,#101014,#101015,#101016,#101017,#101018,#101019,#101020,
#101021,#101022,#101023,#101024,#101025,#101026,#101027,#101028,#101029,
#101030,#101031,#101032,#101033,#101034,#101035,#101036,#101037,#101038,
#101039,#101040,#101041,#101042,#101043,#101044,#101045,#101046,#101047,
#101048),.UNSPECIFIED.,.F.,.F.,(4,2,2,2,2,2,2,2,2,2,2,2,2,2,2,2,2,2,2,2,
2,2,2,2,2,2,2,2,2,2,2,2,2,2,2,2,2,2,2,2,2,2,2,2,2,2,2,4),(0.0026092829850963,
0.0203081228422541,0.0467104773415106,0.0573073440081075,0.0658992178962575,
0.0767494629243784,0.108072536354288,0.132854431634225,0.139607191542061,
0.144557005284787,0.151706565335001,0.183970979646304,0.209620746036483,
0.219934792552778,0.228507886012935,0.239406533000283,0.269303262627802,
0.287812881356171,0.296028645927189,0.302778346521195,0.30767737886147,
0.314632811108762,0.342639844609213,0.372509459836443,0.382881754334163,
0.391370675190917,0.402148795054376,0.42566704672463,0.456307544582424,
0.464617915238406,0.469625184685304,0.475508964095064,0.487990162648659,
0.515911946016534,0.531105983501541,0.543483252563705,0.552143259439136,
0.561701492758515,0.580973981377501,0.61508504263462,0.62302251830787,0.62960410971002,
0.634510358801496,0.641664597586085,0.661399903408521,0.686602160681216,
0.703168776920759,0.71239184097541),.UNSPECIFIED.) ;
#1353=B_SPLINE_CURVE_WITH_KNOTS('',3,(#101052,#101053,#101054,#101055,#101056,
#101057,#101058,#101059,#101060,#101061,#101062,#101063,#101064,#101065,
#101066,#101067,#101068,#101069,#101070,#101071,#101072,#101073,#101074,
#101075,#101076,#101077,#101078,#101079),.UNSPECIFIED.,.F.,.F.,(4,3,3,3,
3,3,3,3,3,4),(34.5575191899869,34.6694625957267,34.7811806864541,34.8927675157327,
35.0042581797606,35.1156876439035,35.2271277908985,35.3385701031107,35.4501056657722,
35.508675576093),.UNSPECIFIED.) ;
#1354=B_SPLINE_CURVE_WITH_KNOTS('',3,(#101080,#101081,#101082,#101083,#101084,
#101085,#101086,#101087,#101088,#101089,#101090,#101091,#101092,#101093,
#101094,#101095,#101096,#101097,#101098,#101099,#101100,#101101,#101102,
#101103,#101104,#101105,#101106,#101107,#101108,#101109,#101110,#101111,
#101112,#101113,#101114,#101115,#101116,#101117,#101118,#101119,#101120,
#101121,#101122,#101123,#101124,#101125,#101126,#101127,#101128,#101129,
#101130,#101131,#101132,#101133,#101134,#101135,#101136,#101137,#101138,
#101139,#101140),.UNSPECIFIED.,.F.,.F.,(4,3,3,3,3,3,3,3,3,3,3,3,3,3,3,3,
3,3,3,3,4),(32.5109076064973,32.5937562294461,32.7036643904514,32.8133952660067,
32.9230275064331,33.0326010843926,33.1421558910857,33.2518087048573,33.3615084504932,
33.4714088639723,33.5653960116618,33.6747987943945,33.7840191138006,33.8931380204768,
34.0021964233412,34.111235146482,34.2203746515072,34.3295618237526,34.4389574443397,
34.5370357938774,34.5575191894876),.UNSPECIFIED.) ;
#1355=B_SPLINE_CURVE_WITH_KNOTS('',3,(#101142,#101143,#101144,#101145,#101146,
#101147,#101148,#101149,#101150,#101151,#101152,#101153,#101154,#101155,
#101156,#101157,#101158,#101159,#101160,#101161,#101162,#101163,#101164,
#101165,#101166,#101167,#101168,#101169,#101170,#101171,#101172,#101173,
#101174,#101175,#101176,#101177,#101178,#101179,#101180,#101181,#101182,
#101183,#101184,#101185,#101186,#101187,#101188,#101189,#101190,#101191,
#101192,#101193,#101194,#101195,#101196,#101197,#101198,#101199,#101200,
#101201,#101202,#101203,#101204,#101205,#101206,#101207,#101208,#101209,
#101210,#101211,#101212,#101213,#101214,#101215,#101216,#101217,#101218,
#101219,#101220,#101221,#101222,#101223,#101224,#101225,#101226),
 .UNSPECIFIED.,.F.,.F.,(4,3,3,3,3,3,3,3,3,3,3,3,3,3,3,3,3,3,3,3,3,3,3,3,
3,3,3,3,4),(-0.37524009580756,-0.357518921288721,-0.353499339011914,-0.330618426268463,
-0.324807985426275,-0.303154818283502,-0.286565543774214,-0.2802937315987,
-0.274975128510897,-0.253676729885043,-0.232669298257941,-0.217166169990548,
-0.20837475042749,-0.204726014152323,-0.184286055371377,-0.17045203706431,
-0.149652213060313,-0.139823936654317,-0.135833669251288,-0.132392599709375,
-0.112098960320059,-0.0918017548146832,-0.0716539883511498,-0.067625436545846,
-0.0641202926150906,-0.0443089210862901,-0.0250693388973895,-0.00603116485857798,
-1.6124231245987E-14),.UNSPECIFIED.) ;
#1356=B_SPLINE_CURVE_WITH_KNOTS('',3,(#101228,#101229,#101230,#101231),
 .UNSPECIFIED.,.F.,.F.,(4,4),(0.,0.0129523452064985),.UNSPECIFIED.) ;
#1357=B_SPLINE_CURVE_WITH_KNOTS('',3,(#101232,#101233,#101234,#101235,#101236,
#101237,#101238,#101239,#101240,#101241,#101242,#101243,#101244,#101245,
#101246,#101247,#101248,#101249,#101250,#101251,#101252,#101253,#101254,
#101255,#101256,#101257,#101258,#101259,#101260,#101261,#101262,#101263,
#101264,#101265,#101266,#101267,#101268,#101269,#101270,#101271,#101272,
#101273,#101274,#101275,#101276,#101277,#101278,#101279,#101280,#101281,
#101282,#101283,#101284,#101285,#101286,#101287,#101288,#101289,#101290,
#101291,#101292,#101293,#101294,#101295,#101296,#101297,#101298,#101299,
#101300,#101301,#101302,#101303,#101304,#101305,#101306,#101307,#101308,
#101309,#101310,#101311,#101312,#101313,#101314,#101315,#101316,#101317,
#101318,#101319),.UNSPECIFIED.,.F.,.F.,(4,3,3,3,3,3,3,3,3,3,3,3,3,3,3,3,
3,3,3,3,3,3,3,3,3,3,3,3,3,4),(-0.38016989466375,-0.360311058062006,-0.358093714841499,
-0.34471487570795,-0.336915355012495,-0.332696989994484,-0.312888599506859,
-0.296964105449495,-0.291611990627701,-0.287054657778508,-0.266573287948675,
-0.246125188667504,-0.230967053262615,-0.222333883223211,-0.217980615396263,
-0.196924263842872,-0.185492647047948,-0.16498333041885,-0.154671872267672,
-0.149608894129304,-0.146454177730597,-0.125463903654776,-0.103990194256974,
-0.0825564409435494,-0.0772771397702884,-0.0730031458537735,-0.0510763331729567,
-0.0292998033466994,-0.007759983282897,0.),.UNSPECIFIED.) ;
#1358=B_SPLINE_CURVE_WITH_KNOTS('',3,(#101445,#101446,#101447,#101448,#101449,
#101450,#101451,#101452,#101453,#101454,#101455,#101456,#101457,#101458,
#101459,#101460,#101461,#101462,#101463,#101464,#101465,#101466,#101467,
#101468,#101469,#101470,#101471,#101472,#101473,#101474,#101475,#101476,
#101477,#101478,#101479,#101480,#101481,#101482,#101483,#101484,#101485,
#101486,#101487,#101488,#101489,#101490,#101491,#101492,#101493,#101494,
#101495,#101496,#101497,#101498,#101499,#101500,#101501,#101502,#101503,
#101504,#101505,#101506,#101507,#101508,#101509,#101510,#101511,#101512,
#101513,#101514,#101515,#101516,#101517,#101518,#101519,#101520,#101521,
#101522,#101523,#101524,#101525,#101526,#101527,#101528,#101529),
 .UNSPECIFIED.,.F.,.F.,(4,3,3,3,3,3,3,3,3,3,3,3,3,3,3,3,3,3,3,3,3,3,3,3,
3,3,3,3,4),(0.,0.0198999736214445,0.022033478855472,0.0414468202729217,
0.0603279893210927,0.0659853869923778,0.0696582620916686,0.0895889830255989,
0.110292888835956,0.130996794646314,0.134529829243006,0.138089195898059,
0.158922736380717,0.179545457140466,0.194222826116571,0.203107891092953,
0.207554446770544,0.227794854702371,0.248829911754691,0.265094672958623,
0.273893002460397,0.277903852040319,0.299536877312563,0.319299235095571,
0.325159379351979,0.330782663134293,0.352647695498619,0.37432272203279,
0.378914100184376),.UNSPECIFIED.) ;
#1359=B_SPLINE_CURVE_WITH_KNOTS('',3,(#101530,#101531,#101532,#101533),
 .UNSPECIFIED.,.F.,.F.,(4,4),(-0.0129525315802166,0.),.UNSPECIFIED.) ;
#1360=B_SPLINE_CURVE_WITH_KNOTS('',3,(#101658,#101659,#101660,#101661,#101662,
#101663,#101664,#101665,#101666,#101667,#101668,#101669,#101670,#101671,
#101672,#101673,#101674,#101675,#101676,#101677,#101678,#101679,#101680,
#101681,#101682,#101683,#101684,#101685,#101686,#101687,#101688,#101689,
#101690,#101691,#101692,#101693,#101694,#101695,#101696,#101697,#101698,
#101699,#101700,#101701,#101702,#101703,#101704,#101705,#101706,#101707,
#101708,#101709,#101710,#101711,#101712,#101713,#101714,#101715,#101716,
#101717,#101718,#101719,#101720,#101721,#101722,#101723,#101724,#101725,
#101726,#101727,#101728,#101729,#101730,#101731,#101732,#101733,#101734,
#101735,#101736,#101737,#101738,#101739,#101740,#101741,#101742),
 .UNSPECIFIED.,.F.,.F.,(4,3,3,3,3,3,3,3,3,3,3,3,3,3,3,3,3,3,3,3,3,3,3,3,
3,3,3,3,4),(0.,0.0215677198000641,0.0255184714855182,0.0472519117233337,
0.0675132036694678,0.0732612703991268,0.077959247140824,0.0994876515331383,
0.120942349766413,0.143042324147911,0.147548760546303,0.151258390489377,
0.172167334932419,0.192451590106119,0.209342247292407,0.217998538466851,
0.222762834145278,0.243196176321172,0.263823362943062,0.278366679408141,
0.287113906024107,0.292333781104599,0.312535580645166,0.329444159149797,
0.335387151529194,0.339362863956405,0.35904267418776,0.378722484419115,
0.380169894663675),.UNSPECIFIED.) ;
#2109=B_SPLINE_SURFACE_WITH_KNOTS('',3,3,((#101320,#101321,#101322,#101323,
#101324,#101325,#101326,#101327,#101328,#101329,#101330,#101331,#101332,
#101333,#101334,#101335,#101336,#101337,#101338,#101339,#101340,#101341,
#101342,#101343,#101344,#101345,#101346,#101347,#101348,#101349,#101350),
(#101351,#101352,#101353,#101354,#101355,#101356,#101357,#101358,#101359,
#101360,#101361,#101362,#101363,#101364,#101365,#101366,#101367,#101368,
#101369,#101370,#101371,#101372,#101373,#101374,#101375,#101376,#101377,
#101378,#101379,#101380,#101381),(#101382,#101383,#101384,#101385,#101386,
#101387,#101388,#101389,#101390,#101391,#101392,#101393,#101394,#101395,
#101396,#101397,#101398,#101399,#101400,#101401,#101402,#101403,#101404,
#101405,#101406,#101407,#101408,#101409,#101410,#101411,#101412),(#101413,
#101414,#101415,#101416,#101417,#101418,#101419,#101420,#101421,#101422,
#101423,#101424,#101425,#101426,#101427,#101428,#101429,#101430,#101431,
#101432,#101433,#101434,#101435,#101436,#101437,#101438,#101439,#101440,
#101441,#101442,#101443)),.UNSPECIFIED.,.F.,.F.,.F.,(4,4),(4,1,1,1,1,1,
1,1,1,1,1,1,1,1,1,1,1,1,1,1,1,1,1,1,1,1,1,1,4),(-0.0003307145317139,0.0332819478446879),
(8.30276167405425,9.27440145626992,10.2460412384856,11.2176810207013,12.1893208029169,
13.1609605851326,14.1326003673483,15.104240149564,16.0758799317796,17.0475197139953,
18.019159496211,18.9907992784267,19.9624390606423,20.934078842858,21.9057186250737,
22.8773584072894,23.848998189505,24.8206379717207,25.7922777539364,26.763917536152,
27.7355573183677,28.7071971005834,29.6788368827991,30.6504766650147,31.6221164472304,
32.5937562294461,33.5653960116618,34.5370357938774,35.5090062906248),
 .UNSPECIFIED.) ;
#2110=B_SPLINE_SURFACE_WITH_KNOTS('',3,3,((#101534,#101535,#101536,#101537,
#101538,#101539,#101540,#101541,#101542,#101543,#101544,#101545,#101546,
#101547,#101548,#101549,#101550,#101551,#101552,#101553,#101554,#101555,
#101556,#101557,#101558,#101559,#101560,#101561,#101562,#101563,#101564),
(#101565,#101566,#101567,#101568,#101569,#101570,#101571,#101572,#101573,
#101574,#101575,#101576,#101577,#101578,#101579,#101580,#101581,#101582,
#101583,#101584,#101585,#101586,#101587,#101588,#101589,#101590,#101591,
#101592,#101593,#101594,#101595),(#101596,#101597,#101598,#101599,#101600,
#101601,#101602,#101603,#101604,#101605,#101606,#101607,#101608,#101609,
#101610,#101611,#101612,#101613,#101614,#101615,#101616,#101617,#101618,
#101619,#101620,#101621,#101622,#101623,#101624,#101625,#101626),(#101627,
#101628,#101629,#101630,#101631,#101632,#101633,#101634,#101635,#101636,
#101637,#101638,#101639,#101640,#101641,#101642,#101643,#101644,#101645,
#101646,#101647,#101648,#101649,#101650,#101651,#101652,#101653,#101654,
#101655,#101656,#101657)),.UNSPECIFIED.,.F.,.F.,.F.,(4,4),(4,1,1,1,1,1,
1,1,1,1,1,1,1,1,1,1,1,1,1,1,1,1,1,1,1,1,1,1,4),(-0.000267659600955013,0.0333309127327678),
(11.6148788829061,12.5868540099704,13.5584937921861,14.5301335744018,15.5017733566174,
16.4734131388331,17.4450529210488,18.4166927032644,19.3883324854801,20.3599722676958,
21.3316120499115,22.3032518321271,23.2748916143428,24.2465313965585,25.2181711787741,
26.1898109609898,27.1614507432055,28.1330905254212,29.1047303076368,30.0763700898525,
31.0480098720682,32.0196496542838,32.9912894364995,33.9629292187152,34.9345690009309,
35.9062087831465,36.8778485653622,37.8494883475779,38.8211281297935),
 .UNSPECIFIED.) ;
#2855=PLANE('',#54039) ;
#2856=PLANE('',#54040) ;
#2857=PLANE('',#54041) ;
#5750=LINE('',#98753,#8964) ;
#5751=LINE('',#98890,#8965) ;
#5752=LINE('',#99178,#8966) ;
#5753=LINE('',#99301,#8967) ;
#8964=VECTOR('',#67253,1.67775) ;
#8965=VECTOR('',#67258,1.67775) ;
#8966=VECTOR('',#67261,1.67775) ;
#8967=VECTOR('',#67264,1.67775) ;
#10486=CYLINDRICAL_SURFACE('',#54028,1.67775) ;
#10487=CYLINDRICAL_SURFACE('',#54030,1.67775) ;
#10488=CYLINDRICAL_SURFACE('',#54031,1.67775) ;
#10489=CYLINDRICAL_SURFACE('',#54032,1.67775) ;
#10490=CYLINDRICAL_SURFACE('',#54033,1.9635) ;
#10491=CYLINDRICAL_SURFACE('',#54037,1.67775) ;
#13223=FACE_OUTER_BOUND('',#16406,.T.) ;
#13224=FACE_OUTER_BOUND('',#16407,.T.) ;
#13225=FACE_OUTER_BOUND('',#16408,.T.) ;
#13226=FACE_OUTER_BOUND('',#16409,.T.) ;
#13227=FACE_OUTER_BOUND('',#16410,.T.) ;
#13228=FACE_OUTER_BOUND('',#16412,.T.) ;
#13229=FACE_OUTER_BOUND('',#16413,.T.) ;
#13230=FACE_OUTER_BOUND('',#16414,.T.) ;
#13231=FACE_OUTER_BOUND('',#16415,.T.) ;
#13232=FACE_OUTER_BOUND('',#16416,.T.) ;
#13233=FACE_OUTER_BOUND('',#16417,.T.) ;
#16406=EDGE_LOOP('',(#42682,#42683,#42684,#42685)) ;
#16407=EDGE_LOOP('',(#42686,#42687,#42688,#42689)) ;
#16408=EDGE_LOOP('',(#42690,#42691,#42692,#42693,#42694,#42695)) ;
#16409=EDGE_LOOP('',(#42696,#42697,#42698,#42699,#42700,#42701)) ;
#16410=EDGE_LOOP('',(#42702,#42703,#42704,#42705,#42706,#42707,#42708,#42709,
#42710,#42711,#42712,#42713,#42714)) ;
#16411=EDGE_LOOP('',(#42715)) ;
#16412=EDGE_LOOP('',(#42716,#42717,#42718,#42719,#42720)) ;
#16413=EDGE_LOOP('',(#42721,#42722,#42723,#42724,#42725)) ;
#16414=EDGE_LOOP('',(#42726,#42727,#42728,#42729,#42730,#42731,#42732,#42733,
#42734,#42735,#42736,#42737,#42738,#42739,#42740,#42741,#42742)) ;
#16415=EDGE_LOOP('',(#42743,#42744,#42745,#42746,#42747,#42748,#42749,#42750,
#42751,#42752,#42753,#42754,#42755,#42756,#42757)) ;
#16416=EDGE_LOOP('',(#42758,#42759,#42760,#42761,#42762)) ;
#16417=EDGE_LOOP('',(#42763)) ;
#19122=CIRCLE('',#54029,1.67775) ;
#19123=CIRCLE('',#54034,1.9635) ;
#19124=CIRCLE('',#54035,1.9635) ;
#19125=CIRCLE('',#54036,1.9635) ;
#19126=CIRCLE('',#54038,1.67775) ;
#23000=VERTEX_POINT('',#98751) ;
#23001=VERTEX_POINT('',#98752) ;
#23002=VERTEX_POINT('',#98754) ;
#23003=VERTEX_POINT('',#98835) ;
#23004=VERTEX_POINT('',#98888) ;
#23005=VERTEX_POINT('',#98889) ;
#23006=VERTEX_POINT('',#99176) ;
#23007=VERTEX_POINT('',#99177) ;
#23008=VERTEX_POINT('',#99179) ;
#23009=VERTEX_POINT('',#99238) ;
#23010=VERTEX_POINT('',#99299) ;
#23011=VERTEX_POINT('',#99300) ;
#23012=VERTEX_POINT('',#99302) ;
#23013=VERTEX_POINT('',#99427) ;
#23014=VERTEX_POINT('',#99535) ;
#23015=VERTEX_POINT('',#99536) ;
#23016=VERTEX_POINT('',#99538) ;
#23017=VERTEX_POINT('',#99547) ;
#23018=VERTEX_POINT('',#99741) ;
#23019=VERTEX_POINT('',#99935) ;
#23020=VERTEX_POINT('',#100132) ;
#23021=VERTEX_POINT('',#100194) ;
#23022=VERTEX_POINT('',#100196) ;
#23023=VERTEX_POINT('',#100202) ;
#23024=VERTEX_POINT('',#100396) ;
#23025=VERTEX_POINT('',#100593) ;
#23026=VERTEX_POINT('',#100787) ;
#23027=VERTEX_POINT('',#100949) ;
#23028=VERTEX_POINT('',#100952) ;
#23029=VERTEX_POINT('',#101049) ;
#23030=VERTEX_POINT('',#101051) ;
#23031=VERTEX_POINT('',#101227) ;
#23032=VERTEX_POINT('',#101444) ;
#29619=EDGE_CURVE('',#23000,#23001,#5750,.T.) ;
#29620=EDGE_CURVE('',#23002,#23000,#1329,.F.) ;
#29621=EDGE_CURVE('',#23003,#23002,#19122,.T.) ;
#29622=EDGE_CURVE('',#23003,#23001,#1330,.T.) ;
#29623=EDGE_CURVE('',#23004,#23005,#5751,.T.) ;
#29624=EDGE_CURVE('',#23000,#23004,#1331,.F.) ;
#29625=EDGE_CURVE('',#23001,#23005,#1332,.T.) ;
#29626=EDGE_CURVE('',#23006,#23007,#5752,.T.) ;
#29627=EDGE_CURVE('',#23008,#23006,#1333,.T.) ;
#29628=EDGE_CURVE('',#23004,#23008,#1334,.F.) ;
#29629=EDGE_CURVE('',#23005,#23009,#1335,.T.) ;
#29630=EDGE_CURVE('',#23009,#23007,#1336,.T.) ;
#29631=EDGE_CURVE('',#23010,#23011,#5753,.T.) ;
#29632=EDGE_CURVE('',#23012,#23010,#1337,.T.) ;
#29633=EDGE_CURVE('',#23006,#23012,#1338,.T.) ;
#29634=EDGE_CURVE('',#23007,#23013,#1339,.T.) ;
#29635=EDGE_CURVE('',#23013,#23011,#1340,.F.) ;
#29636=EDGE_CURVE('',#23014,#23015,#19123,.T.) ;
#29637=EDGE_CURVE('',#23015,#23016,#1341,.T.) ;
#29638=EDGE_CURVE('',#23016,#23017,#1342,.T.) ;
#29639=EDGE_CURVE('',#23017,#23018,#1343,.T.) ;
#29640=EDGE_CURVE('',#23018,#23019,#1344,.T.) ;
#29641=EDGE_CURVE('',#23019,#23020,#1345,.T.) ;
#29642=EDGE_CURVE('',#23021,#23020,#19124,.F.) ;
#29643=EDGE_CURVE('',#23021,#23022,#1346,.T.) ;
#29644=EDGE_CURVE('',#23022,#23023,#1347,.T.) ;
#29645=EDGE_CURVE('',#23023,#23024,#1348,.T.) ;
#29646=EDGE_CURVE('',#23024,#23025,#1349,.T.) ;
#29647=EDGE_CURVE('',#23025,#23026,#1350,.T.) ;
#29648=EDGE_CURVE('',#23026,#23014,#1351,.T.) ;
#29649=EDGE_CURVE('',#23027,#23027,#19125,.T.) ;
#29650=EDGE_CURVE('',#23011,#23028,#1352,.F.) ;
#29651=EDGE_CURVE('',#23029,#23028,#19126,.T.) ;
#29652=EDGE_CURVE('',#23030,#23029,#1353,.T.) ;
#29653=EDGE_CURVE('',#23010,#23030,#1354,.T.) ;
#29654=EDGE_CURVE('',#23014,#23029,#1355,.T.) ;
#29655=EDGE_CURVE('',#23028,#23031,#1356,.T.) ;
#29656=EDGE_CURVE('',#23031,#23015,#1357,.T.) ;
#29657=EDGE_CURVE('',#23032,#23021,#1358,.T.) ;
#29658=EDGE_CURVE('',#23032,#23002,#1359,.T.) ;
#29659=EDGE_CURVE('',#23020,#23003,#1360,.T.) ;
#42682=ORIENTED_EDGE('',*,*,#29619,.F.) ;
#42683=ORIENTED_EDGE('',*,*,#29620,.F.) ;
#42684=ORIENTED_EDGE('',*,*,#29621,.F.) ;
#42685=ORIENTED_EDGE('',*,*,#29622,.T.) ;
#42686=ORIENTED_EDGE('',*,*,#29623,.F.) ;
#42687=ORIENTED_EDGE('',*,*,#29624,.F.) ;
#42688=ORIENTED_EDGE('',*,*,#29619,.T.) ;
#42689=ORIENTED_EDGE('',*,*,#29625,.T.) ;
#42690=ORIENTED_EDGE('',*,*,#29626,.F.) ;
#42691=ORIENTED_EDGE('',*,*,#29627,.F.) ;
#42692=ORIENTED_EDGE('',*,*,#29628,.F.) ;
#42693=ORIENTED_EDGE('',*,*,#29623,.T.) ;
#42694=ORIENTED_EDGE('',*,*,#29629,.T.) ;
#42695=ORIENTED_EDGE('',*,*,#29630,.T.) ;
#42696=ORIENTED_EDGE('',*,*,#29631,.F.) ;
#42697=ORIENTED_EDGE('',*,*,#29632,.F.) ;
#42698=ORIENTED_EDGE('',*,*,#29633,.F.) ;
#42699=ORIENTED_EDGE('',*,*,#29626,.T.) ;
#42700=ORIENTED_EDGE('',*,*,#29634,.T.) ;
#42701=ORIENTED_EDGE('',*,*,#29635,.T.) ;
#42702=ORIENTED_EDGE('',*,*,#29636,.T.) ;
#42703=ORIENTED_EDGE('',*,*,#29637,.T.) ;
#42704=ORIENTED_EDGE('',*,*,#29638,.T.) ;
#42705=ORIENTED_EDGE('',*,*,#29639,.T.) ;
#42706=ORIENTED_EDGE('',*,*,#29640,.T.) ;
#42707=ORIENTED_EDGE('',*,*,#29641,.T.) ;
#42708=ORIENTED_EDGE('',*,*,#29642,.F.) ;
#42709=ORIENTED_EDGE('',*,*,#29643,.T.) ;
#42710=ORIENTED_EDGE('',*,*,#29644,.T.) ;
#42711=ORIENTED_EDGE('',*,*,#29645,.T.) ;
#42712=ORIENTED_EDGE('',*,*,#29646,.T.) ;
#42713=ORIENTED_EDGE('',*,*,#29647,.T.) ;
#42714=ORIENTED_EDGE('',*,*,#29648,.T.) ;
#42715=ORIENTED_EDGE('',*,*,#29649,.F.) ;
#42716=ORIENTED_EDGE('',*,*,#29631,.T.) ;
#42717=ORIENTED_EDGE('',*,*,#29650,.T.) ;
#42718=ORIENTED_EDGE('',*,*,#29651,.F.) ;
#42719=ORIENTED_EDGE('',*,*,#29652,.F.) ;
#42720=ORIENTED_EDGE('',*,*,#29653,.F.) ;
#42721=ORIENTED_EDGE('',*,*,#29636,.F.) ;
#42722=ORIENTED_EDGE('',*,*,#29654,.T.) ;
#42723=ORIENTED_EDGE('',*,*,#29651,.T.) ;
#42724=ORIENTED_EDGE('',*,*,#29655,.T.) ;
#42725=ORIENTED_EDGE('',*,*,#29656,.T.) ;
#42726=ORIENTED_EDGE('',*,*,#29654,.F.) ;
#42727=ORIENTED_EDGE('',*,*,#29648,.F.) ;
#42728=ORIENTED_EDGE('',*,*,#29647,.F.) ;
#42729=ORIENTED_EDGE('',*,*,#29646,.F.) ;
#42730=ORIENTED_EDGE('',*,*,#29645,.F.) ;
#42731=ORIENTED_EDGE('',*,*,#29644,.F.) ;
#42732=ORIENTED_EDGE('',*,*,#29643,.F.) ;
#42733=ORIENTED_EDGE('',*,*,#29657,.F.) ;
#42734=ORIENTED_EDGE('',*,*,#29658,.T.) ;
#42735=ORIENTED_EDGE('',*,*,#29620,.T.) ;
#42736=ORIENTED_EDGE('',*,*,#29624,.T.) ;
#42737=ORIENTED_EDGE('',*,*,#29628,.T.) ;
#42738=ORIENTED_EDGE('',*,*,#29627,.T.) ;
#42739=ORIENTED_EDGE('',*,*,#29633,.T.) ;
#42740=ORIENTED_EDGE('',*,*,#29632,.T.) ;
#42741=ORIENTED_EDGE('',*,*,#29653,.T.) ;
#42742=ORIENTED_EDGE('',*,*,#29652,.T.) ;
#42743=ORIENTED_EDGE('',*,*,#29656,.F.) ;
#42744=ORIENTED_EDGE('',*,*,#29655,.F.) ;
#42745=ORIENTED_EDGE('',*,*,#29650,.F.) ;
#42746=ORIENTED_EDGE('',*,*,#29635,.F.) ;
#42747=ORIENTED_EDGE('',*,*,#29634,.F.) ;
#42748=ORIENTED_EDGE('',*,*,#29630,.F.) ;
#42749=ORIENTED_EDGE('',*,*,#29629,.F.) ;
#42750=ORIENTED_EDGE('',*,*,#29625,.F.) ;
#42751=ORIENTED_EDGE('',*,*,#29622,.F.) ;
#42752=ORIENTED_EDGE('',*,*,#29659,.F.) ;
#42753=ORIENTED_EDGE('',*,*,#29641,.F.) ;
#42754=ORIENTED_EDGE('',*,*,#29640,.F.) ;
#42755=ORIENTED_EDGE('',*,*,#29639,.F.) ;
#42756=ORIENTED_EDGE('',*,*,#29638,.F.) ;
#42757=ORIENTED_EDGE('',*,*,#29637,.F.) ;
#42758=ORIENTED_EDGE('',*,*,#29657,.T.) ;
#42759=ORIENTED_EDGE('',*,*,#29642,.T.) ;
#42760=ORIENTED_EDGE('',*,*,#29659,.T.) ;
#42761=ORIENTED_EDGE('',*,*,#29621,.T.) ;
#42762=ORIENTED_EDGE('',*,*,#29658,.F.) ;
#42763=ORIENTED_EDGE('',*,*,#29649,.T.) ;
#48441=ADVANCED_FACE('',(#13223),#10486,.T.) ;
#48442=ADVANCED_FACE('',(#13224),#10487,.T.) ;
#48443=ADVANCED_FACE('',(#13225),#10488,.T.) ;
#48444=ADVANCED_FACE('',(#13226),#10489,.T.) ;
#48445=ADVANCED_FACE('',(#13227,#761),#10490,.T.) ;
#48446=ADVANCED_FACE('',(#13228),#10491,.T.) ;
#48447=ADVANCED_FACE('',(#13229),#2855,.T.) ;
#48448=ADVANCED_FACE('',(#13230),#2109,.F.) ;
#48449=ADVANCED_FACE('',(#13231),#2110,.F.) ;
#48450=ADVANCED_FACE('',(#13232),#2856,.T.) ;
#48451=ADVANCED_FACE('',(#13233),#2857,.F.) ;
#49074=CLOSED_SHELL('',(#48441,#48442,#48443,#48444,#48445,#48446,#48447,
#48448,#48449,#48450,#48451)) ;
#54027=AXIS2_PLACEMENT_3D('',#98749,#67249,#67250) ;
#54028=AXIS2_PLACEMENT_3D('',#98750,#67251,#67252) ;
#54029=AXIS2_PLACEMENT_3D('',#98836,#67254,#67255) ;
#54030=AXIS2_PLACEMENT_3D('',#98887,#67256,#67257) ;
#54031=AXIS2_PLACEMENT_3D('',#99175,#67259,#67260) ;
#54032=AXIS2_PLACEMENT_3D('',#99298,#67262,#67263) ;
#54033=AXIS2_PLACEMENT_3D('',#99534,#67265,#67266) ;
#54034=AXIS2_PLACEMENT_3D('',#99537,#67267,#67268) ;
#54035=AXIS2_PLACEMENT_3D('',#100195,#67269,#67270) ;
#54036=AXIS2_PLACEMENT_3D('',#100950,#67271,#67272) ;
#54037=AXIS2_PLACEMENT_3D('',#100951,#67273,#67274) ;
#54038=AXIS2_PLACEMENT_3D('',#101050,#67275,#67276) ;
#54039=AXIS2_PLACEMENT_3D('',#101141,#67277,#67278) ;
#54040=AXIS2_PLACEMENT_3D('',#101743,#67279,#67280) ;
#54041=AXIS2_PLACEMENT_3D('',#101744,#67281,#67282) ;
#67249=DIRECTION('axis',(0.,0.,1.)) ;
#67250=DIRECTION('refdir',(1.,0.,0.)) ;
#67251=DIRECTION('center_axis',(0.,-1.,0.)) ;
#67252=DIRECTION('ref_axis',(0.457808359486171,0.,0.889050901796169)) ;
#67253=DIRECTION('',(0.,1.,0.)) ;
#67254=DIRECTION('center_axis',(0.,1.,0.)) ;
#67255=DIRECTION('ref_axis',(-1.,0.,0.)) ;
#67256=DIRECTION('center_axis',(0.,-1.,0.)) ;
#67257=DIRECTION('ref_axis',(0.457808359486171,0.,0.889050901796169)) ;
#67258=DIRECTION('',(0.,1.,0.)) ;
#67259=DIRECTION('center_axis',(0.,-1.,0.)) ;
#67260=DIRECTION('ref_axis',(0.457808359486171,0.,0.889050901796169)) ;
#67261=DIRECTION('',(0.,1.,0.)) ;
#67262=DIRECTION('center_axis',(0.,-1.,0.)) ;
#67263=DIRECTION('ref_axis',(0.457808359486171,0.,0.889050901796169)) ;
#67264=DIRECTION('',(0.,1.,0.)) ;
#67265=DIRECTION('center_axis',(0.,-1.,0.)) ;
#67266=DIRECTION('ref_axis',(-1.,0.,0.)) ;
#67267=DIRECTION('center_axis',(0.,-1.,0.)) ;
#67268=DIRECTION('ref_axis',(-1.,0.,0.)) ;
#67269=DIRECTION('center_axis',(0.,-1.,0.)) ;
#67270=DIRECTION('ref_axis',(-1.,0.,0.)) ;
#67271=DIRECTION('center_axis',(0.,-1.,0.)) ;
#67272=DIRECTION('ref_axis',(-1.,0.,0.)) ;
#67273=DIRECTION('center_axis',(0.,-1.,0.)) ;
#67274=DIRECTION('ref_axis',(0.457808359486171,0.,0.889050901796169)) ;
#67275=DIRECTION('center_axis',(0.,-1.,0.)) ;
#67276=DIRECTION('ref_axis',(-1.,0.,0.)) ;
#67277=DIRECTION('center_axis',(0.,1.,0.)) ;
#67278=DIRECTION('ref_axis',(0.,0.,1.)) ;
#67279=DIRECTION('center_axis',(0.,1.,0.)) ;
#67280=DIRECTION('ref_axis',(-1.,0.,0.)) ;
#67281=DIRECTION('center_axis',(0.,1.,0.)) ;
#67282=DIRECTION('ref_axis',(-1.,0.,0.)) ;
#98749=CARTESIAN_POINT('',(0.,0.,0.)) ;
#98750=CARTESIAN_POINT('Origin',(40.2,265.924309379709,25.0213203435596)) ;
#98751=CARTESIAN_POINT('',(39.4319120248131,264.737243197272,23.5297151931015)) ;
#98752=CARTESIAN_POINT('',(39.4319120325861,264.835792165808,23.5297151890988)) ;
#98753=CARTESIAN_POINT('',(39.4319120248721,265.924309379709,23.5297151930711)) ;
#98754=CARTESIAN_POINT('',(41.1572720979745,265.,26.3991720020989)) ;
#98755=CARTESIAN_POINT('Ctrl Pts',(39.4319120248131,264.737243197272,23.5297151931015)) ;
#98756=CARTESIAN_POINT('Ctrl Pts',(39.4304044404626,264.737322527506,23.5304915094147)) ;
#98757=CARTESIAN_POINT('Ctrl Pts',(39.4288980211696,264.737401933216,23.5312701174534)) ;
#98758=CARTESIAN_POINT('Ctrl Pts',(39.4017655580238,264.738834604452,23.545345971115)) ;
#98759=CARTESIAN_POINT('Ctrl Pts',(39.3764867953982,264.740209382512,23.5592996683641)) ;
#98760=CARTESIAN_POINT('Ctrl Pts',(39.3158646983467,264.743609119489,23.5948338131558)) ;
#98761=CARTESIAN_POINT('Ctrl Pts',(39.2809371147819,264.745656348017,23.6170831411784)) ;
#98762=CARTESIAN_POINT('Ctrl Pts',(39.2049495917101,264.750310835025,23.6695383876079)) ;
#98763=CARTESIAN_POINT('Ctrl Pts',(39.1643713622691,264.752936389273,23.7003689485121)) ;
#98764=CARTESIAN_POINT('Ctrl Pts',(39.0570776606221,264.760235887148,23.7898749823946)) ;
#98765=CARTESIAN_POINT('Ctrl Pts',(38.9935196330723,264.764976767591,23.8520753394917)) ;
#98766=CARTESIAN_POINT('Ctrl Pts',(38.9062589178821,264.771892128461,23.9522005420064)) ;
#98767=CARTESIAN_POINT('Ctrl Pts',(38.8786504561284,264.774150951797,23.9865165132885)) ;
#98768=CARTESIAN_POINT('Ctrl Pts',(38.8405383737826,264.777332483655,24.0379042863935)) ;
#98769=CARTESIAN_POINT('Ctrl Pts',(38.8289405250687,264.778310004615,24.0541393705838)) ;
#98770=CARTESIAN_POINT('Ctrl Pts',(38.8082442588673,264.780066197532,24.0842314407711)) ;
#98771=CARTESIAN_POINT('Ctrl Pts',(38.7990569823385,264.780849756839,24.0980228174524)) ;
#98772=CARTESIAN_POINT('Ctrl Pts',(38.7755205297153,264.782871876341,24.1345146328457)) ;
#98773=CARTESIAN_POINT('Ctrl Pts',(38.7615090530597,264.784091369515,24.1574279566855)) ;
#98774=CARTESIAN_POINT('Ctrl Pts',(38.730302404386,264.786867654561,24.2113270965558)) ;
#98775=CARTESIAN_POINT('Ctrl Pts',(38.7135265532737,264.788407229425,24.2425411933755)) ;
#98776=CARTESIAN_POINT('Ctrl Pts',(38.6474731304393,264.794766372148,24.3753674532139)) ;
#98777=CARTESIAN_POINT('Ctrl Pts',(38.6075300929458,264.799398931744,24.4812875596889)) ;
#98778=CARTESIAN_POINT('Ctrl Pts',(38.5650438565067,264.806558905916,24.6411622330249)) ;
#98779=CARTESIAN_POINT('Ctrl Pts',(38.5539491631154,264.808878661246,24.6925074891467)) ;
#98780=CARTESIAN_POINT('Ctrl Pts',(38.5402808673343,264.812647790166,24.7741479734373)) ;
#98781=CARTESIAN_POINT('Ctrl Pts',(38.536090856418,264.814048948341,24.804138367956)) ;
#98782=CARTESIAN_POINT('Ctrl Pts',(38.5294393775916,264.816857677078,24.8634124000482)) ;
#98783=CARTESIAN_POINT('Ctrl Pts',(38.5269311980604,264.818263301234,24.8926798806991)) ;
#98784=CARTESIAN_POINT('Ctrl Pts',(38.522465377297,264.821931900017,24.9679834005038)) ;
#98785=CARTESIAN_POINT('Ctrl Pts',(38.5216335168716,264.824226849211,25.0140596063819)) ;
#98786=CARTESIAN_POINT('Ctrl Pts',(38.5253565800552,264.832412630974,25.1750513356149)) ;
#98787=CARTESIAN_POINT('Ctrl Pts',(38.5398229695952,264.838550190996,25.2894098581918)) ;
#98788=CARTESIAN_POINT('Ctrl Pts',(38.5789038623145,264.847610943719,25.4574467850682)) ;
#98789=CARTESIAN_POINT('Ctrl Pts',(38.5948222900754,264.850597622558,25.5128122743674)) ;
#98790=CARTESIAN_POINT('Ctrl Pts',(38.6202728864776,264.85449866004,25.5867700258602)) ;
#98791=CARTESIAN_POINT('Ctrl Pts',(38.6273491209682,264.855512885922,25.6061625263056)) ;
#98792=CARTESIAN_POINT('Ctrl Pts',(38.6407241304923,264.857303372889,25.6408170745013)) ;
#98793=CARTESIAN_POINT('Ctrl Pts',(38.6468928931367,264.858085781612,25.6561240611006)) ;
#98794=CARTESIAN_POINT('Ctrl Pts',(38.6632446090061,264.86005640523,25.6950328008638)) ;
#98795=CARTESIAN_POINT('Ctrl Pts',(38.6737456634063,264.861228016883,25.7184956608131)) ;
#98796=CARTESIAN_POINT('Ctrl Pts',(38.6990171899898,264.863862871164,25.7716501225304)) ;
#98797=CARTESIAN_POINT('Ctrl Pts',(38.7141371771553,264.865311673756,25.8011639226423)) ;
#98798=CARTESIAN_POINT('Ctrl Pts',(38.7755726633357,264.870803061255,25.9128015316757)) ;
#98799=CARTESIAN_POINT('Ctrl Pts',(38.8279036513412,264.874703119596,25.9914154149038)) ;
#98800=CARTESIAN_POINT('Ctrl Pts',(38.9278985951457,264.881563118496,26.1172295012224)) ;
#98801=CARTESIAN_POINT('Ctrl Pts',(38.9722858731208,264.884452275983,26.1667355574291)) ;
#98802=CARTESIAN_POINT('Ctrl Pts',(39.0426653094159,264.88892443338,26.2364274694627)) ;
#98803=CARTESIAN_POINT('Ctrl Pts',(39.0665050907615,264.890422153507,26.258695810473)) ;
#98804=CARTESIAN_POINT('Ctrl Pts',(39.1125792981033,264.89329468395,26.2992835698611)) ;
#98805=CARTESIAN_POINT('Ctrl Pts',(39.1346660304974,264.894662773603,26.3177528355227)) ;
#98806=CARTESIAN_POINT('Ctrl Pts',(39.1884456830622,264.897977455058,26.3604215819749)) ;
#98807=CARTESIAN_POINT('Ctrl Pts',(39.2205465973335,264.899943189666,26.38407673626)) ;
#98808=CARTESIAN_POINT('Ctrl Pts',(39.2930597605727,264.904356110779,26.4336252000818)) ;
#98809=CARTESIAN_POINT('Ctrl Pts',(39.3338015852083,264.906818185425,26.4589731084199)) ;
#98810=CARTESIAN_POINT('Ctrl Pts',(39.4559885188033,264.914121405243,26.5279116968206)) ;
#98811=CARTESIAN_POINT('Ctrl Pts',(39.5400108830261,264.919051974656,26.566566029181)) ;
#98812=CARTESIAN_POINT('Ctrl Pts',(39.6713920558248,264.926343153125,26.6143273997752)) ;
#98813=CARTESIAN_POINT('Ctrl Pts',(39.7166702627846,264.928782814097,26.62864443888)) ;
#98814=CARTESIAN_POINT('Ctrl Pts',(39.7817310051742,264.932132170627,26.6462182009804)) ;
#98815=CARTESIAN_POINT('Ctrl Pts',(39.8010567606912,264.933107837232,26.6510707398458)) ;
#98816=CARTESIAN_POINT('Ctrl Pts',(39.8369522698017,264.93487889742,26.6594070004195)) ;
#98817=CARTESIAN_POINT('Ctrl Pts',(39.8534961786273,264.935678613719,26.6629861608072)) ;
#98818=CARTESIAN_POINT('Ctrl Pts',(39.8976837332061,264.937775992996,26.6718481000392)) ;
#98819=CARTESIAN_POINT('Ctrl Pts',(39.9254118456879,264.939052573819,26.6766869163251)) ;
#98820=CARTESIAN_POINT('Ctrl Pts',(39.9907384050409,264.941993744339,26.6864002567276)) ;
#98821=CARTESIAN_POINT('Ctrl Pts',(40.028406633528,264.943638655548,26.690702703065)) ;
#98822=CARTESIAN_POINT('Ctrl Pts',(40.2052785704075,264.951244315129,26.7048543697477)) ;
#98823=CARTESIAN_POINT('Ctrl Pts',(40.3452067720937,264.95697305041,26.6985890791927)) ;
#98824=CARTESIAN_POINT('Ctrl Pts',(40.5176897119491,264.964809821159,26.6690991456072)) ;
#98825=CARTESIAN_POINT('Ctrl Pts',(40.5524325630894,264.966425446333,26.6620192273418)) ;
#98826=CARTESIAN_POINT('Ctrl Pts',(40.6147723482532,264.969404799588,26.6472441009216)) ;
#98827=CARTESIAN_POINT('Ctrl Pts',(40.6424463134638,264.970756548302,26.6399324993173)) ;
#98828=CARTESIAN_POINT('Ctrl Pts',(40.704465240716,264.973856933408,26.6218374269499)) ;
#98829=CARTESIAN_POINT('Ctrl Pts',(40.7386766867003,264.975617437676,26.6106495448928)) ;
#98830=CARTESIAN_POINT('Ctrl Pts',(40.8512779527651,264.981583670503,26.5697730560285)) ;
#98831=CARTESIAN_POINT('Ctrl Pts',(40.9277947283892,264.985928426018,26.5353154878895)) ;
#98832=CARTESIAN_POINT('Ctrl Pts',(41.0550811114644,264.993557678104,26.4661086949452)) ;
#98833=CARTESIAN_POINT('Ctrl Pts',(41.1071118799309,264.996802126154,26.4340211651883)) ;
#98834=CARTESIAN_POINT('Ctrl Pts',(41.1572720979745,265.,26.3991720020989)) ;
#98835=CARTESIAN_POINT('',(39.225659978706,265.,26.3871558334356)) ;
#98836=CARTESIAN_POINT('Origin',(40.2,265.,25.0213203435596)) ;
#98837=CARTESIAN_POINT('Ctrl Pts',(39.225659978706,265.,26.3871558334356)) ;
#98838=CARTESIAN_POINT('Ctrl Pts',(39.2153375643007,264.999398586693,26.3797921783351)) ;
#98839=CARTESIAN_POINT('Ctrl Pts',(39.2050987251971,264.998803540393,26.3723115745025)) ;
#98840=CARTESIAN_POINT('Ctrl Pts',(39.1821482809501,264.997471097196,26.3551413105944)) ;
#98841=CARTESIAN_POINT('Ctrl Pts',(39.1694882714317,264.996737051312,26.3453845773693)) ;
#98842=CARTESIAN_POINT('Ctrl Pts',(39.0582891688161,264.990282099836,26.2571252243299)) ;
#98843=CARTESIAN_POINT('Ctrl Pts',(38.9687388195114,264.985009519897,26.1679316979276)) ;
#98844=CARTESIAN_POINT('Ctrl Pts',(38.8614953736439,264.977536268327,26.0339081445413)) ;
#98845=CARTESIAN_POINT('Ctrl Pts',(38.8344434094844,264.975526916063,25.997119319476)) ;
#98846=CARTESIAN_POINT('Ctrl Pts',(38.7871725793157,264.971727220694,25.9270122319354)) ;
#98847=CARTESIAN_POINT('Ctrl Pts',(38.7665491542183,264.969949584461,25.8940044557118)) ;
#98848=CARTESIAN_POINT('Ctrl Pts',(38.7317053771711,264.96670064448,25.8336643349143)) ;
#98849=CARTESIAN_POINT('Ctrl Pts',(38.7170547799005,264.965243750705,25.806600675999)) ;
#98850=CARTESIAN_POINT('Ctrl Pts',(38.6857195260224,264.961905303656,25.7447082336931)) ;
#98851=CARTESIAN_POINT('Ctrl Pts',(38.669476806028,264.960010976513,25.709676263679)) ;
#98852=CARTESIAN_POINT('Ctrl Pts',(38.6084925735989,264.952175279112,25.5652917050987)) ;
#98853=CARTESIAN_POINT('Ctrl Pts',(38.5741549049405,264.945929659729,25.4519274112468)) ;
#98854=CARTESIAN_POINT('Ctrl Pts',(38.5362429748598,264.935175265875,25.2533264290485)) ;
#98855=CARTESIAN_POINT('Ctrl Pts',(38.5267069951294,264.930709147059,25.1696659586808)) ;
#98856=CARTESIAN_POINT('Ctrl Pts',(38.5225723652007,264.925266877297,25.0618943820493)) ;
#98857=CARTESIAN_POINT('Ctrl Pts',(38.5221659172324,264.924086606359,25.0381315005049)) ;
#98858=CARTESIAN_POINT('Ctrl Pts',(38.5223322482953,264.922134803343,24.9979984297071)) ;
#98859=CARTESIAN_POINT('Ctrl Pts',(38.5226396085222,264.921350945212,24.9816320007903)) ;
#98860=CARTESIAN_POINT('Ctrl Pts',(38.5239062545065,264.919564286199,24.9437381579236)) ;
#98861=CARTESIAN_POINT('Ctrl Pts',(38.5250407417903,264.91856991652,24.9222204106408)) ;
#98862=CARTESIAN_POINT('Ctrl Pts',(38.5348843182911,264.912353275722,24.7856232519015)) ;
#98863=CARTESIAN_POINT('Ctrl Pts',(38.5550341356524,264.907581508538,24.6716697907738)) ;
#98864=CARTESIAN_POINT('Ctrl Pts',(38.608101188325,264.899364401452,24.4858161861708)) ;
#98865=CARTESIAN_POINT('Ctrl Pts',(38.6346609459615,264.896006783232,24.4125354873651)) ;
#98866=CARTESIAN_POINT('Ctrl Pts',(38.6793366403557,264.891034860123,24.3117592553561)) ;
#98867=CARTESIAN_POINT('Ctrl Pts',(38.6933164274786,264.889549493163,24.2825386113984)) ;
#98868=CARTESIAN_POINT('Ctrl Pts',(38.7208594501208,264.886735836765,24.22900592723)) ;
#98869=CARTESIAN_POINT('Ctrl Pts',(38.7341990250379,264.885415421392,24.204591322851)) ;
#98870=CARTESIAN_POINT('Ctrl Pts',(38.7666878401857,264.882288877449,24.1484908820612)) ;
#98871=CARTESIAN_POINT('Ctrl Pts',(38.7862905747062,264.88046722329,24.1170856303193)) ;
#98872=CARTESIAN_POINT('Ctrl Pts',(38.8609217532805,264.873750076278,24.005886153229)) ;
#98873=CARTESIAN_POINT('Ctrl Pts',(38.9217937713385,264.868650688891,23.9302555633882)) ;
#98874=CARTESIAN_POINT('Ctrl Pts',(39.0363356794035,264.859830231537,23.8107666806675)) ;
#98875=CARTESIAN_POINT('Ctrl Pts',(39.0868222911744,264.856153642658,23.7641844678424)) ;
#98876=CARTESIAN_POINT('Ctrl Pts',(39.1622368816876,264.851078579735,23.702717217297)) ;
#98877=CARTESIAN_POINT('Ctrl Pts',(39.1849142564075,264.849601641214,23.6851812929999)) ;
#98878=CARTESIAN_POINT('Ctrl Pts',(39.2265980280825,264.84698943238,23.6546222421566)) ;
#98879=CARTESIAN_POINT('Ctrl Pts',(39.2454445236879,264.845844401979,23.6413931574044)) ;
#98880=CARTESIAN_POINT('Ctrl Pts',(39.2776898373826,264.843953426749,23.6197357915535)) ;
#98881=CARTESIAN_POINT('Ctrl Pts',(39.2909448615541,264.843195393758,23.6111026026035)) ;
#98882=CARTESIAN_POINT('Ctrl Pts',(39.3216635266847,264.841481540571,23.5917082536414)) ;
#98883=CARTESIAN_POINT('Ctrl Pts',(39.3392055457963,264.84053325582,23.5810777732057)) ;
#98884=CARTESIAN_POINT('Ctrl Pts',(39.3815807666403,264.838304021937,23.5564492333377)) ;
#98885=CARTESIAN_POINT('Ctrl Pts',(39.4065800980265,264.837037998039,23.5427596292232)) ;
#98886=CARTESIAN_POINT('Ctrl Pts',(39.4319120325861,264.835792165808,23.5297151890988)) ;
#98887=CARTESIAN_POINT('Origin',(40.2,265.924309379709,25.0213203435596)) ;
#98888=CARTESIAN_POINT('',(39.431912024867,264.240044136826,23.5297151930737)) ;
#98889=CARTESIAN_POINT('',(39.4319120259791,264.338362624254,23.529715192501)) ;
#98890=CARTESIAN_POINT('',(39.4319120248721,265.924309379709,23.5297151930711)) ;
#98891=CARTESIAN_POINT('Ctrl Pts',(39.431912024867,264.240044136826,23.5297151930737)) ;
#98892=CARTESIAN_POINT('Ctrl Pts',(39.4132822099684,264.241024674624,23.5393084401859)) ;
#98893=CARTESIAN_POINT('Ctrl Pts',(39.3948328986984,264.241985998715,23.5492503106463)) ;
#98894=CARTESIAN_POINT('Ctrl Pts',(39.2729335404419,264.24830290277,23.6179164536233)) ;
#98895=CARTESIAN_POINT('Ctrl Pts',(39.1757869152903,264.253187306839,23.687158681559)) ;
#98896=CARTESIAN_POINT('Ctrl Pts',(39.0460663182673,264.260530210574,23.8022047100275)) ;
#98897=CARTESIAN_POINT('Ctrl Pts',(39.007138576516,264.26285881752,23.8402669489468)) ;
#98898=CARTESIAN_POINT('Ctrl Pts',(38.9407781639254,264.267146306372,23.9117854632675)) ;
#98899=CARTESIAN_POINT('Ctrl Pts',(38.912659037804,264.269080067746,23.9445380049841)) ;
#98900=CARTESIAN_POINT('Ctrl Pts',(38.8677636804408,264.272397320149,24.0011064082021)) ;
#98901=CARTESIAN_POINT('Ctrl Pts',(38.8502881123139,264.273753733266,24.0243410122428)) ;
#98902=CARTESIAN_POINT('Ctrl Pts',(38.8153418670443,264.276611452506,24.0734075775326)) ;
#98903=CARTESIAN_POINT('Ctrl Pts',(38.7979701382822,264.278115593169,24.099296009554)) ;
#98904=CARTESIAN_POINT('Ctrl Pts',(38.7500244828146,264.282521456516,24.1752382698391)) ;
#98905=CARTESIAN_POINT('Ctrl Pts',(38.7213423528314,264.285485033205,24.2264275700949)) ;
#98906=CARTESIAN_POINT('Ctrl Pts',(38.6420784451439,264.294733748247,24.3870887329753)) ;
#98907=CARTESIAN_POINT('Ctrl Pts',(38.6005604560298,264.301221827089,24.5005900581633)) ;
#98908=CARTESIAN_POINT('Ctrl Pts',(38.5650399790021,264.308842703721,24.6438489225981)) ;
#98909=CARTESIAN_POINT('Ctrl Pts',(38.5591580175469,264.310225385382,24.6702980604476)) ;
#98910=CARTESIAN_POINT('Ctrl Pts',(38.5496071397796,264.312701315645,24.7187552541532)) ;
#98911=CARTESIAN_POINT('Ctrl Pts',(38.5457316795646,264.31380222938,24.7407162895493)) ;
#98912=CARTESIAN_POINT('Ctrl Pts',(38.5397820767606,264.315670306164,24.7788592795642)) ;
#98913=CARTESIAN_POINT('Ctrl Pts',(38.5375042501585,264.316446941494,24.7950045600758)) ;
#98914=CARTESIAN_POINT('Ctrl Pts',(38.5325424462824,264.318304447274,24.8343078218836)) ;
#98915=CARTESIAN_POINT('Ctrl Pts',(38.530105103436,264.31937333216,24.8574926834839)) ;
#98916=CARTESIAN_POINT('Ctrl Pts',(38.5204609114229,264.324559288927,24.9721711131197)) ;
#98917=CARTESIAN_POINT('Ctrl Pts',(38.5202859549722,264.328406459296,25.0641045598926)) ;
#98918=CARTESIAN_POINT('Ctrl Pts',(38.535639344848,264.336486444213,25.2553265917216)) ;
#98919=CARTESIAN_POINT('Ctrl Pts',(38.552551418043,264.340713029794,25.3541369107347)) ;
#98920=CARTESIAN_POINT('Ctrl Pts',(38.5870709941029,264.346753498454,25.4844786072675)) ;
#98921=CARTESIAN_POINT('Ctrl Pts',(38.5970218535698,264.34833978593,25.5178245528935)) ;
#98922=CARTESIAN_POINT('Ctrl Pts',(38.6169652688593,264.351278999889,25.5777848005739)) ;
#98923=CARTESIAN_POINT('Ctrl Pts',(38.6266112524308,264.352620737927,25.6045007513464)) ;
#98924=CARTESIAN_POINT('Ctrl Pts',(38.6500147219436,264.355712330818,25.6645056491577)) ;
#98925=CARTESIAN_POINT('Ctrl Pts',(38.6641750930185,264.357474497521,25.6976215509824)) ;
#98926=CARTESIAN_POINT('Ctrl Pts',(38.7254323492215,264.364697130764,25.8290137118034)) ;
#98927=CARTESIAN_POINT('Ctrl Pts',(38.7809825392229,264.370421352668,25.9230426007967)) ;
#98928=CARTESIAN_POINT('Ctrl Pts',(38.8940442842774,264.380544138254,26.0778087351502)) ;
#98929=CARTESIAN_POINT('Ctrl Pts',(38.947717807763,264.384909042365,26.1409090739036)) ;
#98930=CARTESIAN_POINT('Ctrl Pts',(39.0211926660056,264.390145964443,26.2153625111654)) ;
#98931=CARTESIAN_POINT('Ctrl Pts',(39.0368591779498,264.391224519625,26.2306287977629)) ;
#98932=CARTESIAN_POINT('Ctrl Pts',(39.0647325093007,264.393071082758,26.2567471035433)) ;
#98933=CARTESIAN_POINT('Ctrl Pts',(39.0768061899353,264.393847731681,26.2677340974336)) ;
#98934=CARTESIAN_POINT('Ctrl Pts',(39.1068853402126,264.395727852864,26.2943138828354)) ;
#98935=CARTESIAN_POINT('Ctrl Pts',(39.1250655496236,264.396818345749,26.3097023653233)) ;
#98936=CARTESIAN_POINT('Ctrl Pts',(39.1964886378161,264.400954621437,26.3675931609585)) ;
#98937=CARTESIAN_POINT('Ctrl Pts',(39.2519762097907,264.403861845856,26.4072271333079)) ;
#98938=CARTESIAN_POINT('Ctrl Pts',(39.3795119909923,264.410221069298,26.4870706366956)) ;
#98939=CARTESIAN_POINT('Ctrl Pts',(39.4524225757243,264.413654975052,26.5255650883706)) ;
#98940=CARTESIAN_POINT('Ctrl Pts',(39.5640618021591,264.41891785501,26.5743781619071)) ;
#98941=CARTESIAN_POINT('Ctrl Pts',(39.6008076241019,264.420649696972,26.5889217806131)) ;
#98942=CARTESIAN_POINT('Ctrl Pts',(39.6710580311562,264.423987279655,26.6138950077881)) ;
#98943=CARTESIAN_POINT('Ctrl Pts',(39.7044430811037,264.425584314431,26.6245972430872)) ;
#98944=CARTESIAN_POINT('Ctrl Pts',(39.7654369931549,264.428533855109,26.6420628957595)) ;
#98945=CARTESIAN_POINT('Ctrl Pts',(39.7929293845093,264.429874692,26.6491854573395)) ;
#98946=CARTESIAN_POINT('Ctrl Pts',(39.8553889502476,264.432950917972,26.663685905923)) ;
#98947=CARTESIAN_POINT('Ctrl Pts',(39.8904369731581,264.434698100471,26.6706510933627)) ;
#98948=CARTESIAN_POINT('Ctrl Pts',(40.0361795808214,264.442052870894,26.6948058301963)) ;
#98949=CARTESIAN_POINT('Ctrl Pts',(40.1482254517613,264.447943435313,26.7020062253947)) ;
#98950=CARTESIAN_POINT('Ctrl Pts',(40.3389737752404,264.4580232707,26.6951645407568)) ;
#98951=CARTESIAN_POINT('Ctrl Pts',(40.4175163670847,264.46218041606,26.686780079503)) ;
#98952=CARTESIAN_POINT('Ctrl Pts',(40.5173846668642,264.467270170071,26.6689309757283)) ;
#98953=CARTESIAN_POINT('Ctrl Pts',(40.5395072172764,264.468384663882,26.6645150242635)) ;
#98954=CARTESIAN_POINT('Ctrl Pts',(40.5774537599682,264.470266194265,26.6561412732288)) ;
#98955=CARTESIAN_POINT('Ctrl Pts',(40.5933198664014,264.471043199999,26.6523967767594)) ;
#98956=CARTESIAN_POINT('Ctrl Pts',(40.6314711798773,264.472888883523,26.6428037197553)) ;
#98957=CARTESIAN_POINT('Ctrl Pts',(40.6536946027953,264.473946118853,26.6367264888121)) ;
#98958=CARTESIAN_POINT('Ctrl Pts',(40.766709351244,264.479261796876,26.6033050080665)) ;
#98959=CARTESIAN_POINT('Ctrl Pts',(40.8551963966758,264.483228683936,26.5687554680522)) ;
#98960=CARTESIAN_POINT('Ctrl Pts',(41.0298470370369,264.491427195233,26.4828802114617)) ;
#98961=CARTESIAN_POINT('Ctrl Pts',(41.1152876456138,264.495651183807,26.4309480136934)) ;
#98962=CARTESIAN_POINT('Ctrl Pts',(41.2230008839063,264.501660112862,26.3515357254904)) ;
#98963=CARTESIAN_POINT('Ctrl Pts',(41.2497771271807,264.50321532966,26.330507716289)) ;
#98964=CARTESIAN_POINT('Ctrl Pts',(41.2977182226069,264.506126255737,26.2904415791122)) ;
#98965=CARTESIAN_POINT('Ctrl Pts',(41.3190739450083,264.507472200388,26.2716512592455)) ;
#98966=CARTESIAN_POINT('Ctrl Pts',(41.366592257236,264.510585991811,26.2276482170967)) ;
#98967=CARTESIAN_POINT('Ctrl Pts',(41.3924336290613,264.512366659027,26.2021108568985)) ;
#98968=CARTESIAN_POINT('Ctrl Pts',(41.4806720200064,264.518766764598,26.1090579451391)) ;
#98969=CARTESIAN_POINT('Ctrl Pts',(41.5383253186715,264.523559098989,26.0372811396274)) ;
#98970=CARTESIAN_POINT('Ctrl Pts',(41.6272172466736,264.531931248712,25.9058293430199)) ;
#98971=CARTESIAN_POINT('Ctrl Pts',(41.6612921986356,264.535473596637,25.8483213590859)) ;
#98972=CARTESIAN_POINT('Ctrl Pts',(41.710035790308,264.540988151677,25.7535887779138)) ;
#98973=CARTESIAN_POINT('Ctrl Pts',(41.7269617821315,264.543013082286,25.7176056491031)) ;
#98974=CARTESIAN_POINT('Ctrl Pts',(41.7499024725837,264.545897277305,25.6639654953731)) ;
#98975=CARTESIAN_POINT('Ctrl Pts',(41.7569264164679,264.546802836909,25.6467567131915)) ;
#98976=CARTESIAN_POINT('Ctrl Pts',(41.7699110786407,264.548517063275,25.613368819403)) ;
#98977=CARTESIAN_POINT('Ctrl Pts',(41.7759110196701,264.549327494081,25.5972080622188)) ;
#98978=CARTESIAN_POINT('Ctrl Pts',(41.7920540946538,264.551568457438,25.551584084156)) ;
#98979=CARTESIAN_POINT('Ctrl Pts',(41.8016274932276,264.552971018738,25.5219254149515)) ;
#98980=CARTESIAN_POINT('Ctrl Pts',(41.8228040228152,264.55630328929,25.4494751076159)) ;
#98981=CARTESIAN_POINT('Ctrl Pts',(41.8335482285678,264.558204348483,25.4064565310586)) ;
#98982=CARTESIAN_POINT('Ctrl Pts',(41.8695547832027,264.565706673534,25.2333912928301)) ;
#98983=CARTESIAN_POINT('Ctrl Pts',(41.8810828186049,264.571165169789,25.1009902504229)) ;
#98984=CARTESIAN_POINT('Ctrl Pts',(41.8758237428878,264.578660469262,24.9336764807616)) ;
#98985=CARTESIAN_POINT('Ctrl Pts',(41.873634363284,264.580253280481,24.8987867066433)) ;
#98986=CARTESIAN_POINT('Ctrl Pts',(41.8676951768917,264.583198191272,24.8357302838891)) ;
#98987=CARTESIAN_POINT('Ctrl Pts',(41.8643165202015,264.584538787246,24.8075417638774)) ;
#98988=CARTESIAN_POINT('Ctrl Pts',(41.8550632610952,264.58761867794,24.7440254752234)) ;
#98989=CARTESIAN_POINT('Ctrl Pts',(41.8487695766841,264.589369925801,24.7087735509979)) ;
#98990=CARTESIAN_POINT('Ctrl Pts',(41.8240241960479,264.595318019672,24.5919164116561)) ;
#98991=CARTESIAN_POINT('Ctrl Pts',(41.8006007087929,264.599653780808,24.5114993901129)) ;
#98992=CARTESIAN_POINT('Ctrl Pts',(41.7329485687108,264.609811759641,24.3307620720685)) ;
#98993=CARTESIAN_POINT('Ctrl Pts',(41.6846948181059,264.615663167122,24.2323431382963)) ;
#98994=CARTESIAN_POINT('Ctrl Pts',(41.6160022054311,264.622198068891,24.1211886820815)) ;
#98995=CARTESIAN_POINT('Ctrl Pts',(41.6044536027076,264.623248136182,24.1032738269612)) ;
#98996=CARTESIAN_POINT('Ctrl Pts',(41.5834555221782,264.62506743693,24.0720244323337)) ;
#98997=CARTESIAN_POINT('Ctrl Pts',(41.5741477893204,264.625844237799,24.0586003501734)) ;
#98998=CARTESIAN_POINT('Ctrl Pts',(41.5506661607752,264.62773407751,24.0257685578035)) ;
#98999=CARTESIAN_POINT('Ctrl Pts',(41.5362690012208,264.628833716756,24.0065259354761)) ;
#99000=CARTESIAN_POINT('Ctrl Pts',(41.5028997471058,264.631268735791,23.9638682052474)) ;
#99001=CARTESIAN_POINT('Ctrl Pts',(41.4837000904252,264.632592705322,23.940641396621)) ;
#99002=CARTESIAN_POINT('Ctrl Pts',(41.4142081997694,264.637169513495,23.8610405469919)) ;
#99003=CARTESIAN_POINT('Ctrl Pts',(41.3607441122175,264.640320386567,23.8075557090152)) ;
#99004=CARTESIAN_POINT('Ctrl Pts',(41.2428899909118,264.646926019045,23.7045897054797)) ;
#99005=CARTESIAN_POINT('Ctrl Pts',(41.1781510925646,264.650379714059,23.6558100322662)) ;
#99006=CARTESIAN_POINT('Ctrl Pts',(41.0797837925954,264.655605844451,23.5922885177305)) ;
#99007=CARTESIAN_POINT('Ctrl Pts',(41.0487957146746,264.657248258095,23.5736680687358)) ;
#99008=CARTESIAN_POINT('Ctrl Pts',(40.9924157507406,264.660243250267,23.5422227349849)) ;
#99009=CARTESIAN_POINT('Ctrl Pts',(40.9672532232408,264.66158215339,23.5290151346424)) ;
#99010=CARTESIAN_POINT('Ctrl Pts',(40.9106414927648,264.664604027441,23.5011104865597)) ;
#99011=CARTESIAN_POINT('Ctrl Pts',(40.8790476778546,264.666296895613,23.4867378648453)) ;
#99012=CARTESIAN_POINT('Ctrl Pts',(40.8111312142302,264.669951340191,23.4583495278672)) ;
#99013=CARTESIAN_POINT('Ctrl Pts',(40.7747207640723,264.671919560343,23.4445975041175)) ;
#99014=CARTESIAN_POINT('Ctrl Pts',(40.6626260181984,264.677995338667,23.4066588082306)) ;
#99015=CARTESIAN_POINT('Ctrl Pts',(40.5856752245792,264.682193475733,23.3865701767195)) ;
#99016=CARTESIAN_POINT('Ctrl Pts',(40.436182653323,264.69022147364,23.3586898815297)) ;
#99017=CARTESIAN_POINT('Ctrl Pts',(40.3639757429192,264.694042185173,23.3500228266856)) ;
#99018=CARTESIAN_POINT('Ctrl Pts',(40.2676673315645,264.698897927437,23.3447665557978)) ;
#99019=CARTESIAN_POINT('Ctrl Pts',(40.2438773685744,264.700077716064,23.3439753141406)) ;
#99020=CARTESIAN_POINT('Ctrl Pts',(40.2037374834939,264.70202636514,23.3434949258404)) ;
#99021=CARTESIAN_POINT('Ctrl Pts',(40.1873956270982,264.702807550702,23.343538092777)) ;
#99022=CARTESIAN_POINT('Ctrl Pts',(40.1491056524484,264.704609046989,23.3441987754075)) ;
#99023=CARTESIAN_POINT('Ctrl Pts',(40.1271647404408,264.705620103466,23.3450082926165)) ;
#99024=CARTESIAN_POINT('Ctrl Pts',(40.0787947145311,264.707813825624,23.3477444692676)) ;
#99025=CARTESIAN_POINT('Ctrl Pts',(40.0523824381001,264.708988460367,23.3498670588905)) ;
#99026=CARTESIAN_POINT('Ctrl Pts',(39.9124685060611,264.715135293397,23.3644536531822)) ;
#99027=CARTESIAN_POINT('Ctrl Pts',(39.8004078164719,264.719813436412,23.3878546495737)) ;
#99028=CARTESIAN_POINT('Ctrl Pts',(39.6308878195355,264.727426599087,23.441759169475)) ;
#99029=CARTESIAN_POINT('Ctrl Pts',(39.5713392483099,264.730206995592,23.4645008237095)) ;
#99030=CARTESIAN_POINT('Ctrl Pts',(39.4857769654096,264.734451992723,23.5028882824064)) ;
#99031=CARTESIAN_POINT('Ctrl Pts',(39.458661104631,264.735835640365,23.5159410072526)) ;
#99032=CARTESIAN_POINT('Ctrl Pts',(39.4319120248131,264.737243197272,23.5297151931015)) ;
#99033=CARTESIAN_POINT('Ctrl Pts',(39.4319120325861,264.835792165808,23.5297151890988)) ;
#99034=CARTESIAN_POINT('Ctrl Pts',(39.4603130231985,264.834395396468,23.5150903675857)) ;
#99035=CARTESIAN_POINT('Ctrl Pts',(39.4891320894357,264.833023970378,23.5012765080419)) ;
#99036=CARTESIAN_POINT('Ctrl Pts',(39.621570495771,264.826858751005,23.4423873974807)) ;
#99037=CARTESIAN_POINT('Ctrl Pts',(39.7291763356068,264.822200486286,23.4070294341609)) ;
#99038=CARTESIAN_POINT('Ctrl Pts',(39.8842993407464,264.815252428622,23.3729027993618)) ;
#99039=CARTESIAN_POINT('Ctrl Pts',(39.9294613400335,264.813206303652,23.3648917271524)) ;
#99040=CARTESIAN_POINT('Ctrl Pts',(40.0042188785895,264.809750539146,23.3547698362209)) ;
#99041=CARTESIAN_POINT('Ctrl Pts',(40.0336436247803,264.80837321832,23.3515759696404)) ;
#99042=CARTESIAN_POINT('Ctrl Pts',(40.0938902713359,264.805512382131,23.346644876479)) ;
#99043=CARTESIAN_POINT('Ctrl Pts',(40.1247063534128,264.80402738775,23.3449767284515)) ;
#99044=CARTESIAN_POINT('Ctrl Pts',(40.2108238312162,264.79981339099,23.3426943365568)) ;
#99045=CARTESIAN_POINT('Ctrl Pts',(40.2661325005939,264.797032125976,23.3439628524623)) ;
#99046=CARTESIAN_POINT('Ctrl Pts',(40.4429878790381,264.787926671349,23.356780185482)) ;
#99047=CARTESIAN_POINT('Ctrl Pts',(40.5633658102133,264.781377829567,23.3788528396579)) ;
#99048=CARTESIAN_POINT('Ctrl Pts',(40.7063805511062,264.773686075272,23.4215810446935)) ;
#99049=CARTESIAN_POINT('Ctrl Pts',(40.7322879160633,264.772298066013,23.4300137198069)) ;
#99050=CARTESIAN_POINT('Ctrl Pts',(40.7791251017808,264.769811925624,23.446530855956)) ;
#99051=CARTESIAN_POINT('Ctrl Pts',(40.800120174473,264.768706209724,23.4544113881442)) ;
#99052=CARTESIAN_POINT('Ctrl Pts',(40.8362633101766,264.76682556862,23.4688108536214)) ;
#99053=CARTESIAN_POINT('Ctrl Pts',(40.851483365359,264.766041334621,23.4751359512571)) ;
#99054=CARTESIAN_POINT('Ctrl Pts',(40.888518374427,264.764151098008,23.4911708431225)) ;
#99055=CARTESIAN_POINT('Ctrl Pts',(40.9102232976851,264.763057847776,23.5011236426734)) ;
#99056=CARTESIAN_POINT('Ctrl Pts',(40.9955037482383,264.758793901546,23.5424543974849)) ;
#99057=CARTESIAN_POINT('Ctrl Pts',(41.0572788774782,264.755773936296,23.5773865053189)) ;
#99058=CARTESIAN_POINT('Ctrl Pts',(41.1842684508533,264.749369082032,23.6602265354854)) ;
#99059=CARTESIAN_POINT('Ctrl Pts',(41.2486038687719,264.745997193338,23.709150240806)) ;
#99060=CARTESIAN_POINT('Ctrl Pts',(41.3386056518523,264.740810417845,23.7884530375364)) ;
#99061=CARTESIAN_POINT('Ctrl Pts',(41.367125024726,264.739088619342,23.815416701166)) ;
#99062=CARTESIAN_POINT('Ctrl Pts',(41.4192001521303,264.735765413338,23.8682303681528)) ;
#99063=CARTESIAN_POINT('Ctrl Pts',(41.4429442138599,264.734172386311,23.8938652471206)) ;
#99064=CARTESIAN_POINT('Ctrl Pts',(41.4845884313122,264.731220466203,23.941741214141)) ;
#99065=CARTESIAN_POINT('Ctrl Pts',(41.5027543924094,264.729872808872,23.9637337448904)) ;
#99066=CARTESIAN_POINT('Ctrl Pts',(41.542686176494,264.726765690045,24.0146677451005)) ;
#99067=CARTESIAN_POINT('Ctrl Pts',(41.5640928940294,264.72499379652,24.0438716416054)) ;
#99068=CARTESIAN_POINT('Ctrl Pts',(41.6451194781059,264.717845173489,24.162262436959)) ;
#99069=CARTESIAN_POINT('Ctrl Pts',(41.6970671897372,264.712216355083,24.2563784368131)) ;
#99070=CARTESIAN_POINT('Ctrl Pts',(41.7726258393592,264.702176429026,24.4309190604384)) ;
#99071=CARTESIAN_POINT('Ctrl Pts',(41.7998905682313,264.697798948963,24.5093853963317)) ;
#99072=CARTESIAN_POINT('Ctrl Pts',(41.8269843148759,264.692522927052,24.6111187923016)) ;
#99073=CARTESIAN_POINT('Ctrl Pts',(41.8322978041528,264.69142116348,24.6328010561549)) ;
#99074=CARTESIAN_POINT('Ctrl Pts',(41.840743339365,264.68955193272,24.6705034265262)) ;
#99075=CARTESIAN_POINT('Ctrl Pts',(41.8440769041963,264.68877497752,24.6864735370434)) ;
#99076=CARTESIAN_POINT('Ctrl Pts',(41.8516103411319,264.686916620463,24.7253938146691)) ;
#99077=CARTESIAN_POINT('Ctrl Pts',(41.8555653851039,264.685847238276,24.7483870612886)) ;
#99078=CARTESIAN_POINT('Ctrl Pts',(41.8726082846781,264.680692367483,24.8615479673583)) ;
#99079=CARTESIAN_POINT('Ctrl Pts',(41.8788168598765,264.676873277867,24.9526023552605)) ;
#99080=CARTESIAN_POINT('Ctrl Pts',(41.8762354274784,264.668732611059,25.1459720532812)) ;
#99081=CARTESIAN_POINT('Ctrl Pts',(41.8655238894694,264.664416106255,25.247885381978)) ;
#99082=CARTESIAN_POINT('Ctrl Pts',(41.8389445883439,264.658296193339,25.381699872939)) ;
#99083=CARTESIAN_POINT('Ctrl Pts',(41.8312650486601,264.656736342656,25.4150041386367)) ;
#99084=CARTESIAN_POINT('Ctrl Pts',(41.8153805605958,264.653828810208,25.4754025433758)) ;
#99085=CARTESIAN_POINT('Ctrl Pts',(41.8074966132296,264.652491396902,25.5025682277791)) ;
#99086=CARTESIAN_POINT('Ctrl Pts',(41.7881107364794,264.649416647595,25.5635612135233)) ;
#99087=CARTESIAN_POINT('Ctrl Pts',(41.7762076459389,264.647667319931,25.5972457749204)) ;
#99088=CARTESIAN_POINT('Ctrl Pts',(41.7242087669127,264.640527830177,25.7306769532635)) ;
#99089=CARTESIAN_POINT('Ctrl Pts',(41.6756475536358,264.634881110729,25.826838112927)) ;
#99090=CARTESIAN_POINT('Ctrl Pts',(41.5731002289919,264.624736771575,25.9890891145264)) ;
#99091=CARTESIAN_POINT('Ctrl Pts',(41.5226386536462,264.620273227177,26.0569888497496)) ;
#99092=CARTESIAN_POINT('Ctrl Pts',(41.4530424827636,264.61495654656,26.1372062136278)) ;
#99093=CARTESIAN_POINT('Ctrl Pts',(41.4384921327174,264.613885614521,26.1533336187894)) ;
#99094=CARTESIAN_POINT('Ctrl Pts',(41.4124914762296,264.612048485124,26.1810507607281)) ;
#99095=CARTESIAN_POINT('Ctrl Pts',(41.4011792400443,264.611273842635,26.1927633327704)) ;
#99096=CARTESIAN_POINT('Ctrl Pts',(41.3729105993807,264.609396025964,26.221192237276)) ;
#99097=CARTESIAN_POINT('Ctrl Pts',(41.3557660205301,264.608305895794,26.2377153605269)) ;
#99098=CARTESIAN_POINT('Ctrl Pts',(41.2874091321541,264.604119692389,26.3008438626757)) ;
#99099=CARTESIAN_POINT('Ctrl Pts',(41.2336807478188,264.601167399177,26.3446284719447)) ;
#99100=CARTESIAN_POINT('Ctrl Pts',(41.1110338868682,264.594792418617,26.4325357656551)) ;
#99101=CARTESIAN_POINT('Ctrl Pts',(41.0412867671059,264.591385591186,26.4751938007185)) ;
#99102=CARTESIAN_POINT('Ctrl Pts',(40.9203326320714,264.585506290501,26.5375421574317)) ;
#99103=CARTESIAN_POINT('Ctrl Pts',(40.8707700140226,264.583105984336,26.5601103565535)) ;
#99104=CARTESIAN_POINT('Ctrl Pts',(40.7917355077343,264.579236596979,26.5915536526393)) ;
#99105=CARTESIAN_POINT('Ctrl Pts',(40.762966958361,264.577820168485,26.602095983878)) ;
#99106=CARTESIAN_POINT('Ctrl Pts',(40.7060743851184,264.574996367666,26.6211943892502)) ;
#99107=CARTESIAN_POINT('Ctrl Pts',(40.6779822082692,264.573591504773,26.6298106691421)) ;
#99108=CARTESIAN_POINT('Ctrl Pts',(40.605942498399,264.569958271771,26.6498524155158)) ;
#99109=CARTESIAN_POINT('Ctrl Pts',(40.5617326040619,264.567699651743,26.6602392238709)) ;
#99110=CARTESIAN_POINT('Ctrl Pts',(40.4077286260042,264.55973973429,26.6898863430483)) ;
#99111=CARTESIAN_POINT('Ctrl Pts',(40.2964784955942,264.553808444423,26.6999959491021)) ;
#99112=CARTESIAN_POINT('Ctrl Pts',(40.1248447572972,264.544784897535,26.6984676370998)) ;
#99113=CARTESIAN_POINT('Ctrl Pts',(40.0646970353294,264.541652596257,26.6946898039301)) ;
#99114=CARTESIAN_POINT('Ctrl Pts',(39.9838245097663,264.537582747174,26.6852201651987)) ;
#99115=CARTESIAN_POINT('Ctrl Pts',(39.9628171150925,264.536538795369,26.6823558073586)) ;
#99116=CARTESIAN_POINT('Ctrl Pts',(39.9257030715583,264.534724539274,26.6765767966)) ;
#99117=CARTESIAN_POINT('Ctrl Pts',(39.9095760907824,264.53394692403,26.6738235070944)) ;
#99118=CARTESIAN_POINT('Ctrl Pts',(39.8696445966425,264.532046240274,26.6664035075601)) ;
#99119=CARTESIAN_POINT('Ctrl Pts',(39.8458968326235,264.530936982642,26.6614558124951)) ;
#99120=CARTESIAN_POINT('Ctrl Pts',(39.7925136757706,264.528475268262,26.6491201725161)) ;
#99121=CARTESIAN_POINT('Ctrl Pts',(39.7629557074293,264.527134618253,26.6414344785844)) ;
#99122=CARTESIAN_POINT('Ctrl Pts',(39.6588766295046,264.522445373623,26.6113157674762)) ;
#99123=CARTESIAN_POINT('Ctrl Pts',(39.585723532054,264.519203595309,26.5845110293359)) ;
#99124=CARTESIAN_POINT('Ctrl Pts',(39.4432954874348,264.512611116293,26.5207741953414)) ;
#99125=CARTESIAN_POINT('Ctrl Pts',(39.3742228625323,264.509266863713,26.4838710657085)) ;
#99126=CARTESIAN_POINT('Ctrl Pts',(39.2775358603165,264.504168994166,26.4231752013845)) ;
#99127=CARTESIAN_POINT('Ctrl Pts',(39.2477154412045,264.50253484944,26.4030913255179)) ;
#99128=CARTESIAN_POINT('Ctrl Pts',(39.195531686536,264.499548785321,26.3654538655108)) ;
#99129=CARTESIAN_POINT('Ctrl Pts',(39.1729256258476,264.49821018945,26.3482602951387)) ;
#99130=CARTESIAN_POINT('Ctrl Pts',(39.123576760158,264.495181241812,26.3087100639991)) ;
#99131=CARTESIAN_POINT('Ctrl Pts',(39.0970728033448,264.493480709015,26.2860775029034)) ;
#99132=CARTESIAN_POINT('Ctrl Pts',(38.9945795044098,264.48660028113,26.1928822537341)) ;
#99133=CARTESIAN_POINT('Ctrl Pts',(38.9245044953552,264.481180935281,26.1161732244024)) ;
#99134=CARTESIAN_POINT('Ctrl Pts',(38.8090997805529,264.471080171141,25.9636153183496)) ;
#99135=CARTESIAN_POINT('Ctrl Pts',(38.7617893960508,264.466435593155,25.889695244031)) ;
#99136=CARTESIAN_POINT('Ctrl Pts',(38.7093853084934,264.460844498925,25.7916873838573)) ;
#99137=CARTESIAN_POINT('Ctrl Pts',(38.698738630309,264.45968010146,25.7707280645133)) ;
#99138=CARTESIAN_POINT('Ctrl Pts',(38.6814588642479,264.457748574458,25.7348633958412)) ;
#99139=CARTESIAN_POINT('Ctrl Pts',(38.6745968727737,264.456969632151,25.7200736731255)) ;
#99140=CARTESIAN_POINT('Ctrl Pts',(38.6589425213988,264.455163891134,25.6850035039807)) ;
#99141=CARTESIAN_POINT('Ctrl Pts',(38.6503334909669,264.454146701536,25.6646455180901)) ;
#99142=CARTESIAN_POINT('Ctrl Pts',(38.6128535320748,264.449578247998,25.5708935327125)) ;
#99143=CARTESIAN_POINT('Ctrl Pts',(38.5887756351206,264.446230653195,25.495685692654)) ;
#99144=CARTESIAN_POINT('Ctrl Pts',(38.5431902214919,264.438119819372,25.3088775489508)) ;
#99145=CARTESIAN_POINT('Ctrl Pts',(38.527545539298,264.433382372799,25.1962558630923)) ;
#99146=CARTESIAN_POINT('Ctrl Pts',(38.5220753660632,264.426723565329,25.0473800794649)) ;
#99147=CARTESIAN_POINT('Ctrl Pts',(38.52190005134,264.425105200611,25.0118045253802)) ;
#99148=CARTESIAN_POINT('Ctrl Pts',(38.523617589027,264.42213595683,24.9478897960574)) ;
#99149=CARTESIAN_POINT('Ctrl Pts',(38.5250990081268,264.420797742369,24.9195530196465)) ;
#99150=CARTESIAN_POINT('Ctrl Pts',(38.5300218334654,264.417754200358,24.8562366540208)) ;
#99151=CARTESIAN_POINT('Ctrl Pts',(38.5338452361228,264.416038116422,24.8213008734254)) ;
#99152=CARTESIAN_POINT('Ctrl Pts',(38.5443140332504,264.412319708539,24.7472354394495)) ;
#99153=CARTESIAN_POINT('Ctrl Pts',(38.5512565474712,264.410310104689,24.7081697300542)) ;
#99154=CARTESIAN_POINT('Ctrl Pts',(38.5770222585659,264.403993916823,24.5880707347812)) ;
#99155=CARTESIAN_POINT('Ctrl Pts',(38.600489603566,264.399587895727,24.5081662162692)) ;
#99156=CARTESIAN_POINT('Ctrl Pts',(38.6533425799269,264.391672101551,24.3677383347004)) ;
#99157=CARTESIAN_POINT('Ctrl Pts',(38.6806261169513,264.388164971409,24.3066017974438)) ;
#99158=CARTESIAN_POINT('Ctrl Pts',(38.7224727803526,264.383598086447,24.226131541578)) ;
#99159=CARTESIAN_POINT('Ctrl Pts',(38.7339063112038,264.382417670293,24.205243563097)) ;
#99160=CARTESIAN_POINT('Ctrl Pts',(38.7539170821872,264.380469650882,24.170464653071)) ;
#99161=CARTESIAN_POINT('Ctrl Pts',(38.7622587906277,264.379689647803,24.1564437760821)) ;
#99162=CARTESIAN_POINT('Ctrl Pts',(38.7822466189683,264.377894252709,24.1239365818474)) ;
#99163=CARTESIAN_POINT('Ctrl Pts',(38.7940514362987,264.376887962902,24.1055523714472)) ;
#99164=CARTESIAN_POINT('Ctrl Pts',(38.8530918967326,264.372084294171,24.0174397741805)) ;
#99165=CARTESIAN_POINT('Ctrl Pts',(38.9051766140087,264.368523315023,23.951099699316)) ;
#99166=CARTESIAN_POINT('Ctrl Pts',(39.0343108391942,264.360459630191,23.8099228822857)) ;
#99167=CARTESIAN_POINT('Ctrl Pts',(39.1139941225095,264.355970492159,23.7380024453812)) ;
#99168=CARTESIAN_POINT('Ctrl Pts',(39.2290182103572,264.349577494941,23.6526176660407)) ;
#99169=CARTESIAN_POINT('Ctrl Pts',(39.2587413067597,264.347934487787,23.6320095358068)) ;
#99170=CARTESIAN_POINT('Ctrl Pts',(39.3129535812011,264.344939764203,23.5969607922664)) ;
#99171=CARTESIAN_POINT('Ctrl Pts',(39.3371879240245,264.343601780697,23.5821515940277)) ;
#99172=CARTESIAN_POINT('Ctrl Pts',(39.3848560024173,264.340967349072,23.5546593021696)) ;
#99173=CARTESIAN_POINT('Ctrl Pts',(39.4082380990316,264.339673930004,23.5419058574188)) ;
#99174=CARTESIAN_POINT('Ctrl Pts',(39.4319120259791,264.338362624254,23.529715192501)) ;
#99175=CARTESIAN_POINT('Origin',(40.2,265.924309379709,25.0213203435596)) ;
#99176=CARTESIAN_POINT('',(39.4328938139748,263.738513013137,23.5316344567886)) ;
#99177=CARTESIAN_POINT('',(39.4307622574477,263.837133669222,23.5274649509199)) ;
#99178=CARTESIAN_POINT('',(39.4319120248721,265.924309379709,23.5297151930711)) ;
#99179=CARTESIAN_POINT('',(41.879903193355,264.075690031382,25.0205900571519)) ;
#99180=CARTESIAN_POINT('Ctrl Pts',(41.879903193355,264.075690031382,25.0205900571519)) ;
#99181=CARTESIAN_POINT('Ctrl Pts',(41.8770846065361,264.052182781784,25.5146053170057)) ;
#99182=CARTESIAN_POINT('Ctrl Pts',(41.3905535149138,264.002901986479,26.5550998150335)) ;
#99183=CARTESIAN_POINT('Ctrl Pts',(39.6433242486872,263.927847645466,26.9070374174888)) ;
#99184=CARTESIAN_POINT('Ctrl Pts',(38.3288170683365,263.850527008344,25.6250544739862)) ;
#99185=CARTESIAN_POINT('Ctrl Pts',(38.5878625678462,263.787415464234,24.1488945231714)) ;
#99186=CARTESIAN_POINT('Ctrl Pts',(39.2151105892869,263.750077465832,23.6430887984231)) ;
#99187=CARTESIAN_POINT('Ctrl Pts',(39.4328938139748,263.738513013137,23.5316344567886)) ;
#99188=CARTESIAN_POINT('Ctrl Pts',(41.8777498633429,264.076929005015,25.0206431782745)) ;
#99189=CARTESIAN_POINT('Ctrl Pts',(41.8777408662402,264.078070021636,24.9983518880119)) ;
#99190=CARTESIAN_POINT('Ctrl Pts',(41.8772876117826,264.079198153112,24.9760620559688)) ;
#99191=CARTESIAN_POINT('Ctrl Pts',(41.8756533446456,264.081220516053,24.9354943906631)) ;
#99192=CARTESIAN_POINT('Ctrl Pts',(41.8746170375289,264.082120366858,24.9172143808539)) ;
#99193=CARTESIAN_POINT('Ctrl Pts',(41.8721313117513,264.083767802207,24.8832235652733)) ;
#99194=CARTESIAN_POINT('Ctrl Pts',(41.8707592432701,264.084518571302,24.8675106546475)) ;
#99195=CARTESIAN_POINT('Ctrl Pts',(41.8668054817143,264.086353342435,24.8285762481613)) ;
#99196=CARTESIAN_POINT('Ctrl Pts',(41.8639600573264,264.08742444931,24.8053855863338)) ;
#99197=CARTESIAN_POINT('Ctrl Pts',(41.8481007558253,264.092439213825,24.6952186002258)) ;
#99198=CARTESIAN_POINT('Ctrl Pts',(41.8287452869014,264.096136679526,24.6092893517415)) ;
#99199=CARTESIAN_POINT('Ctrl Pts',(41.7722795253813,264.104180656384,24.4268486715436)) ;
#99200=CARTESIAN_POINT('Ctrl Pts',(41.7328184553478,264.10852135451,24.3314468380638)) ;
#99201=CARTESIAN_POINT('Ctrl Pts',(41.6685406991477,264.114702193171,24.2092476071826)) ;
#99202=CARTESIAN_POINT('Ctrl Pts',(41.6512538387103,264.116299371156,24.1787433330275)) ;
#99203=CARTESIAN_POINT('Ctrl Pts',(41.6182574671597,264.119249025379,24.1245499417344)) ;
#99204=CARTESIAN_POINT('Ctrl Pts',(41.6028772742757,264.120589825226,24.1006756578644)) ;
#99205=CARTESIAN_POINT('Ctrl Pts',(41.5667979621182,264.123665755724,24.0476754475527)) ;
#99206=CARTESIAN_POINT('Ctrl Pts',(41.5457598571171,264.125412671503,24.0187979080923)) ;
#99207=CARTESIAN_POINT('Ctrl Pts',(41.4549745219419,264.132769691326,23.9021950659991)) ;
#99208=CARTESIAN_POINT('Ctrl Pts',(41.3774533465819,264.13866311733,23.8209033826338)) ;
#99209=CARTESIAN_POINT('Ctrl Pts',(41.2318740816957,264.148792620793,23.6960109892401)) ;
#99210=CARTESIAN_POINT('Ctrl Pts',(41.1676963262942,264.152996445767,23.6484495257852)) ;
#99211=CARTESIAN_POINT('Ctrl Pts',(41.0816883045609,264.158103861994,23.5937485473334)) ;
#99212=CARTESIAN_POINT('Ctrl Pts',(41.0627673445744,264.159196823552,23.5822344906057)) ;
#99213=CARTESIAN_POINT('Ctrl Pts',(41.029524355229,264.161057195035,23.5628963825955)) ;
#99214=CARTESIAN_POINT('Ctrl Pts',(41.015307448192,264.161833781896,23.5549012695639)) ;
#99215=CARTESIAN_POINT('Ctrl Pts',(40.9803399299826,264.163699045892,23.5359025094847)) ;
#99216=CARTESIAN_POINT('Ctrl Pts',(40.9594712309489,264.164775394716,23.5251251389604)) ;
#99217=CARTESIAN_POINT('Ctrl Pts',(40.8586337779497,264.169832982762,23.4757026084012)) ;
#99218=CARTESIAN_POINT('Ctrl Pts',(40.7759013935589,264.17356384224,23.4430071403936)) ;
#99219=CARTESIAN_POINT('Ctrl Pts',(40.5927346483632,264.181631738491,23.3869527782545)) ;
#99220=CARTESIAN_POINT('Ctrl Pts',(40.4919549105143,264.185963532902,23.3659779228706)) ;
#99221=CARTESIAN_POINT('Ctrl Pts',(40.3553579648656,264.192123080523,23.3504171927164)) ;
#99222=CARTESIAN_POINT('Ctrl Pts',(40.3207072523946,264.193708113994,23.3475572154833)) ;
#99223=CARTESIAN_POINT('Ctrl Pts',(40.2576288981572,264.196646194499,23.3443198461683)) ;
#99224=CARTESIAN_POINT('Ctrl Pts',(40.229232546643,264.197988111777,23.3435846362962)) ;
#99225=CARTESIAN_POINT('Ctrl Pts',(40.164785572145,264.201081811222,23.3435526711184)) ;
#99226=CARTESIAN_POINT('Ctrl Pts',(40.1287495864773,264.20284597214,23.3446964844213)) ;
#99227=CARTESIAN_POINT('Ctrl Pts',(39.9844645051002,264.210049869502,23.3539362095259)) ;
#99228=CARTESIAN_POINT('Ctrl Pts',(39.877088242865,264.215750719623,23.3713661918496)) ;
#99229=CARTESIAN_POINT('Ctrl Pts',(39.6939907851638,264.22575168644,23.4196539621261)) ;
#99230=CARTESIAN_POINT('Ctrl Pts',(39.6174091990998,264.230018104946,23.4458934499466)) ;
#99231=CARTESIAN_POINT('Ctrl Pts',(39.521990308725,264.23522524435,23.4865011317105)) ;
#99232=CARTESIAN_POINT('Ctrl Pts',(39.5011497412199,264.236355173688,23.4958776010857)) ;
#99233=CARTESIAN_POINT('Ctrl Pts',(39.4657827943611,264.238251990946,23.5126667075724)) ;
#99234=CARTESIAN_POINT('Ctrl Pts',(39.4511624035582,264.239029419329,23.5198700474164)) ;
#99235=CARTESIAN_POINT('Ctrl Pts',(39.4350678387167,264.2398779681,23.5280933016812)) ;
#99236=CARTESIAN_POINT('Ctrl Pts',(39.4334892848808,264.239961121345,23.5289029979362)) ;
#99237=CARTESIAN_POINT('Ctrl Pts',(39.431912024867,264.240044136826,23.5297151930737)) ;
#99238=CARTESIAN_POINT('',(41.8766931555041,264.174309021491,25.0225048790946)) ;
#99239=CARTESIAN_POINT('Ctrl Pts',(39.4319120259791,264.338362624254,23.529715192501)) ;
#99240=CARTESIAN_POINT('Ctrl Pts',(39.4390323455915,264.337968227664,23.5260486512172)) ;
#99241=CARTESIAN_POINT('Ctrl Pts',(39.4461790647084,264.337572220708,23.5224330192047)) ;
#99242=CARTESIAN_POINT('Ctrl Pts',(39.4881142715112,264.335247709388,23.5015931799167)) ;
#99243=CARTESIAN_POINT('Ctrl Pts',(39.5234643057111,264.333284461677,23.4855302747096)) ;
#99244=CARTESIAN_POINT('Ctrl Pts',(39.6323798394147,264.327234989789,23.4405299568904)) ;
#99245=CARTESIAN_POINT('Ctrl Pts',(39.7074593016282,264.323059053107,23.4155515735615)) ;
#99246=CARTESIAN_POINT('Ctrl Pts',(39.855014449483,264.315017525861,23.377787200928)) ;
#99247=CARTESIAN_POINT('Ctrl Pts',(39.9271325458305,264.311161464821,23.3642866306841)) ;
#99248=CARTESIAN_POINT('Ctrl Pts',(40.0235188989513,264.306274048564,23.3527086080441)) ;
#99249=CARTESIAN_POINT('Ctrl Pts',(40.047191066422,264.305095036168,23.3503744339759)) ;
#99250=CARTESIAN_POINT('Ctrl Pts',(40.0871757529087,264.303148234703,23.3472886718005)) ;
#99251=CARTESIAN_POINT('Ctrl Pts',(40.1034628591235,264.302368107889,23.3462704995395)) ;
#99252=CARTESIAN_POINT('Ctrl Pts',(40.1416222774926,264.300570885418,23.3444434898145)) ;
#99253=CARTESIAN_POINT('Ctrl Pts',(40.1634998155945,264.29956295695,23.3438246638934)) ;
#99254=CARTESIAN_POINT('Ctrl Pts',(40.2715341343524,264.294670555204,23.3428834726316)) ;
#99255=CARTESIAN_POINT('Ctrl Pts',(40.3576211551497,264.291033812052,23.3487697908435)) ;
#99256=CARTESIAN_POINT('Ctrl Pts',(40.5463488981929,264.282997093703,23.3763819182621)) ;
#99257=CARTESIAN_POINT('Ctrl Pts',(40.6481730119896,264.278607696969,23.4011600096864)) ;
#99258=CARTESIAN_POINT('Ctrl Pts',(40.7810203141091,264.272339445258,23.4469780031944)) ;
#99259=CARTESIAN_POINT('Ctrl Pts',(40.8146308924844,264.270706451648,23.4597931830893)) ;
#99260=CARTESIAN_POINT('Ctrl Pts',(40.8740092967406,264.267722593989,23.4846474263884)) ;
#99261=CARTESIAN_POINT('Ctrl Pts',(40.8999322062344,264.266385048693,23.4962803503998)) ;
#99262=CARTESIAN_POINT('Ctrl Pts',(40.9564609679694,264.263385806754,23.5233926346267)) ;
#99263=CARTESIAN_POINT('Ctrl Pts',(40.9869122583999,264.261714946371,23.5391632958224)) ;
#99264=CARTESIAN_POINT('Ctrl Pts',(41.1030265753594,264.25512278373,23.6038860112563)) ;
#99265=CARTESIAN_POINT('Ctrl Pts',(41.1847823354294,264.249986467621,23.6594183399636)) ;
#99266=CARTESIAN_POINT('Ctrl Pts',(41.3350220989899,264.239752654803,23.7821033048645)) ;
#99267=CARTESIAN_POINT('Ctrl Pts',(41.4035945727203,264.234681606571,23.8485903103051)) ;
#99268=CARTESIAN_POINT('Ctrl Pts',(41.4812296826987,264.228737573453,23.9378888544084)) ;
#99269=CARTESIAN_POINT('Ctrl Pts',(41.4959517193035,264.22760058577,23.9555424472142)) ;
#99270=CARTESIAN_POINT('Ctrl Pts',(41.5204818627628,264.2256970093,23.9862173857321)) ;
#99271=CARTESIAN_POINT('Ctrl Pts',(41.5304705487348,264.224919610418,23.9990881570199)) ;
#99272=CARTESIAN_POINT('Ctrl Pts',(41.5538499053762,264.223094235373,24.0301366777674)) ;
#99273=CARTESIAN_POINT('Ctrl Pts',(41.5670637864611,264.222056804688,24.0484424923686)) ;
#99274=CARTESIAN_POINT('Ctrl Pts',(41.5955869111078,264.219791557552,24.0896860986495)) ;
#99275=CARTESIAN_POINT('Ctrl Pts',(41.6107083322645,264.218572743293,24.1127460192723)) ;
#99276=CARTESIAN_POINT('Ctrl Pts',(41.6583652766146,264.214637365794,24.1894823813251)) ;
#99277=CARTESIAN_POINT('Ctrl Pts',(41.688459220635,264.211996099433,24.2446135903258)) ;
#99278=CARTESIAN_POINT('Ctrl Pts',(41.7579401169828,264.205177029998,24.3908474717832)) ;
#99279=CARTESIAN_POINT('Ctrl Pts',(41.7924640147267,264.200998968375,24.4839839739778)) ;
#99280=CARTESIAN_POINT('Ctrl Pts',(41.8279961132188,264.194976787318,24.6141867910252)) ;
#99281=CARTESIAN_POINT('Ctrl Pts',(41.8363196099233,264.193349201256,24.6490475845156)) ;
#99282=CARTESIAN_POINT('Ctrl Pts',(41.8492284357439,264.190370997022,24.7119704403943)) ;
#99283=CARTESIAN_POINT('Ctrl Pts',(41.8542288453068,264.189033464771,24.739933402068)) ;
#99284=CARTESIAN_POINT('Ctrl Pts',(41.8625899506186,264.186383643453,24.7946764261395)) ;
#99285=CARTESIAN_POINT('Ctrl Pts',(41.8660190550052,264.185073856958,24.8214373290495)) ;
#99286=CARTESIAN_POINT('Ctrl Pts',(41.8748052654834,264.180879547383,24.9061658870588)) ;
#99287=CARTESIAN_POINT('Ctrl Pts',(41.8777915094445,264.17792889845,24.9643312464074)) ;
#99288=CARTESIAN_POINT('Ctrl Pts',(41.8777495642464,264.174918096163,25.0225295461999)) ;
#99289=CARTESIAN_POINT('Ctrl Pts',(41.8766931555041,264.174309021491,25.0225048790946)) ;
#99290=CARTESIAN_POINT('Ctrl Pts',(41.8779055444877,264.16603034488,25.1973496541196)) ;
#99291=CARTESIAN_POINT('Ctrl Pts',(41.7737573850774,264.13197812256,25.9151209251136)) ;
#99292=CARTESIAN_POINT('Ctrl Pts',(40.7566757434656,264.072152354534,26.9070373909177)) ;
#99293=CARTESIAN_POINT('Ctrl Pts',(38.9566882099319,263.994831717412,26.5444728956893)) ;
#99294=CARTESIAN_POINT('Ctrl Pts',(38.2410020294161,263.91751108029,24.8535549132323)) ;
#99295=CARTESIAN_POINT('Ctrl Pts',(38.9159323185171,263.864945064226,23.8034612485711)) ;
#99296=CARTESIAN_POINT('Ctrl Pts',(39.4117048817585,263.83815259387,23.5372014183592)) ;
#99297=CARTESIAN_POINT('Ctrl Pts',(39.4307622574477,263.837133669222,23.5274649509199)) ;
#99298=CARTESIAN_POINT('Origin',(40.2,265.924309379709,25.0213203435596)) ;
#99299=CARTESIAN_POINT('',(39.4319120248721,263.238554795302,23.5297151930711)) ;
#99300=CARTESIAN_POINT('',(39.4319120248721,263.338461000729,23.5297151930711)) ;
#99301=CARTESIAN_POINT('',(39.4319120248721,265.924309379709,23.5297151930711)) ;
#99302=CARTESIAN_POINT('',(41.8775578586602,263.575690620291,25.0217527388377)) ;
#99303=CARTESIAN_POINT('Ctrl Pts',(41.8777499442681,263.575690620291,25.0217527883483)) ;
#99304=CARTESIAN_POINT('Ctrl Pts',(41.8777329243011,263.572573203823,25.0877849139014)) ;
#99305=CARTESIAN_POINT('Ctrl Pts',(41.8738133493319,263.569455787356,25.1537158423017)) ;
#99306=CARTESIAN_POINT('Ctrl Pts',(41.8660523250862,263.566338370888,25.2190947417381)) ;
#99307=CARTESIAN_POINT('Ctrl Pts',(41.8582740066163,263.563214007747,25.2846193277889)) ;
#99308=CARTESIAN_POINT('Ctrl Pts',(41.8466372278417,263.560089644607,25.3495890519222)) ;
#99309=CARTESIAN_POINT('Ctrl Pts',(41.8312540968924,263.556965281466,25.4135640610002)) ;
#99310=CARTESIAN_POINT('Ctrl Pts',(41.8158157329821,263.553829700334,25.4777687716389)) ;
#99311=CARTESIAN_POINT('Ctrl Pts',(41.7966042220182,263.550694119202,25.5409712531395)) ;
#99312=CARTESIAN_POINT('Ctrl Pts',(41.7737816615251,263.54755853807,25.6027464733022)) ;
#99313=CARTESIAN_POINT('Ctrl Pts',(41.7584624988814,263.545453845332,25.6442117876479)) ;
#99314=CARTESIAN_POINT('Ctrl Pts',(41.7415173929883,263.543349152593,25.68503446504)) ;
#99315=CARTESIAN_POINT('Ctrl Pts',(41.7230070307806,263.541244459855,25.7250920726685)) ;
#99316=CARTESIAN_POINT('Ctrl Pts',(41.6973518096356,263.538327371737,25.7806116119791)) ;
#99317=CARTESIAN_POINT('Ctrl Pts',(41.6686081706387,263.53541028362,25.8348317573898)) ;
#99318=CARTESIAN_POINT('Ctrl Pts',(41.6369308169397,263.532493195502,25.8873889839276)) ;
#99319=CARTESIAN_POINT('Ctrl Pts',(41.6053058407034,263.529580930694,25.9398593088198)) ;
#99320=CARTESIAN_POINT('Ctrl Pts',(41.5707570426465,263.526668665886,25.9906717442065)) ;
#99321=CARTESIAN_POINT('Ctrl Pts',(41.533485809679,263.523756401078,26.0394856827284)) ;
#99322=CARTESIAN_POINT('Ctrl Pts',(41.4962490219902,263.520846827723,26.0882545084494)) ;
#99323=CARTESIAN_POINT('Ctrl Pts',(41.4562950939316,263.517937254367,26.1350280980593)) ;
#99324=CARTESIAN_POINT('Ctrl Pts',(41.4138687824863,263.515027681012,26.1794946143)) ;
#99325=CARTESIAN_POINT('Ctrl Pts',(41.3714662976345,263.512119741672,26.2239361581695)) ;
#99326=CARTESIAN_POINT('Ctrl Pts',(41.3265945328691,263.509211802332,26.2660728326465)) ;
#99327=CARTESIAN_POINT('Ctrl Pts',(41.2795372911181,263.506303862991,26.3056272771177)) ;
#99328=CARTESIAN_POINT('Ctrl Pts',(41.2324894161032,263.503396502476,26.3451738482833)) ;
#99329=CARTESIAN_POINT('Ctrl Pts',(41.1832573162042,263.50048914196,26.382138884622)) ;
#99330=CARTESIAN_POINT('Ctrl Pts',(41.1321587541967,263.497581781445,26.4162845436287)) ;
#99331=CARTESIAN_POINT('Ctrl Pts',(41.0810169293498,263.494671959398,26.4504591122193)) ;
#99332=CARTESIAN_POINT('Ctrl Pts',(41.0280059065627,263.491762137352,26.4818092506801)) ;
#99333=CARTESIAN_POINT('Ctrl Pts',(40.9734723809854,263.488852315306,26.5101405269104)) ;
#99334=CARTESIAN_POINT('Ctrl Pts',(40.918916921347,263.485941322894,26.5384831983319)) ;
#99335=CARTESIAN_POINT('Ctrl Pts',(40.8628382000286,263.483030330481,26.5638043759017)) ;
#99336=CARTESIAN_POINT('Ctrl Pts',(40.8056047559154,263.480119338068,26.5859570241065)) ;
#99337=CARTESIAN_POINT('Ctrl Pts',(40.7482693995172,263.47720316222,26.6081491182511)) ;
#99338=CARTESIAN_POINT('Ctrl Pts',(40.6897756947109,263.474286986371,26.627161250375)) ;
#99339=CARTESIAN_POINT('Ctrl Pts',(40.6305084602919,263.471370810523,26.6428959748877)) ;
#99340=CARTESIAN_POINT('Ctrl Pts',(40.5800585567212,263.46888848126,26.6562898061025)) ;
#99341=CARTESIAN_POINT('Ctrl Pts',(40.5290485721046,263.466406151996,26.6673096974672)) ;
#99342=CARTESIAN_POINT('Ctrl Pts',(40.4777199314581,263.463923822733,26.675925040208)) ;
#99343=CARTESIAN_POINT('Ctrl Pts',(40.4174066934933,263.461006985005,26.6860484179232)) ;
#99344=CARTESIAN_POINT('Ctrl Pts',(40.3564248957029,263.458090147277,26.6928889412897)) ;
#99345=CARTESIAN_POINT('Ctrl Pts',(40.2951619462482,263.455173309549,26.6963693776139)) ;
#99346=CARTESIAN_POINT('Ctrl Pts',(40.2340001096249,263.452261285982,26.6998440695727)) ;
#99347=CARTESIAN_POINT('Ctrl Pts',(40.1725585453303,263.449349262416,26.6999696590415)) ;
#99348=CARTESIAN_POINT('Ctrl Pts',(40.1112320620376,263.446437238849,26.6967203900231)) ;
#99349=CARTESIAN_POINT('Ctrl Pts',(40.0499621389294,263.443527900983,26.6934741177403)) ;
#99350=CARTESIAN_POINT('Ctrl Pts',(39.9888075904029,263.440618563117,26.6868591846697)) ;
#99351=CARTESIAN_POINT('Ctrl Pts',(39.9281639212254,263.437709225252,26.6769018754621)) ;
#99352=CARTESIAN_POINT('Ctrl Pts',(39.867554185143,263.434801515302,26.6669501378552)) ;
#99353=CARTESIAN_POINT('Ctrl Pts',(39.807455260742,263.431893805353,26.65365981585)) ;
#99354=CARTESIAN_POINT('Ctrl Pts',(39.7482561967113,263.428986095404,26.6371088812991)) ;
#99355=CARTESIAN_POINT('Ctrl Pts',(39.689068785836,263.426078957829,26.6205612047491)) ;
#99356=CARTESIAN_POINT('Ctrl Pts',(39.6307813714153,263.423171820254,26.6007543272832)) ;
#99357=CARTESIAN_POINT('Ctrl Pts',(39.5737695135502,263.420264682678,26.5778165498964)) ;
#99358=CARTESIAN_POINT('Ctrl Pts',(39.5167091539581,263.417355071912,26.5548592586425)) ;
#99359=CARTESIAN_POINT('Ctrl Pts',(39.4609269909413,263.414445461146,26.5287659339765)) ;
#99360=CARTESIAN_POINT('Ctrl Pts',(39.4067790474548,263.411535850381,26.4997132490294)) ;
#99361=CARTESIAN_POINT('Ctrl Pts',(39.3526092092718,263.408625063115,26.4706488166421)) ;
#99362=CARTESIAN_POINT('Ctrl Pts',(39.3000753427169,263.405714275849,26.4386229010154)) ;
#99363=CARTESIAN_POINT('Ctrl Pts',(39.249506641468,263.402803488583,26.4038569390559)) ;
#99364=CARTESIAN_POINT('Ctrl Pts',(39.1988476703477,263.399887505289,26.3690289165958)) ;
#99365=CARTESIAN_POINT('Ctrl Pts',(39.1501612777587,263.396971521996,26.3314513835271)) ;
#99366=CARTESIAN_POINT('Ctrl Pts',(39.1037448806965,263.394055538702,26.2913871827066)) ;
#99367=CARTESIAN_POINT('Ctrl Pts',(39.0642028868813,263.391571421005,26.2572566064162)) ;
#99368=CARTESIAN_POINT('Ctrl Pts',(39.0263078400301,263.389087303308,26.2213221902367)) ;
#99369=CARTESIAN_POINT('Ctrl Pts',(38.9902214910315,263.386603185611,26.1837664806937)) ;
#99370=CARTESIAN_POINT('Ctrl Pts',(38.9478786271104,263.383688380968,26.1396995040455)) ;
#99371=CARTESIAN_POINT('Ctrl Pts',(38.9078655732094,263.380773576325,26.0932316296736)) ;
#99372=CARTESIAN_POINT('Ctrl Pts',(38.8704644770455,263.377858771682,26.0446386497097)) ;
#99373=CARTESIAN_POINT('Ctrl Pts',(38.8331252898328,263.374948791831,25.9961261042982)) ;
#99374=CARTESIAN_POINT('Ctrl Pts',(38.798389782311,263.37203881198,25.9454958379628)) ;
#99375=CARTESIAN_POINT('Ctrl Pts',(38.7665017994721,263.369128832129,25.8930588201586)) ;
#99376=CARTESIAN_POINT('Ctrl Pts',(38.7346432991151,263.366221542741,25.8406702837349)) ;
#99377=CARTESIAN_POINT('Ctrl Pts',(38.7056273667572,263.363314253352,25.7864787394361)) ;
#99378=CARTESIAN_POINT('Ctrl Pts',(38.679655286762,263.360406963964,25.730825111288)) ;
#99379=CARTESIAN_POINT('Ctrl Pts',(38.6536977585997,263.357501303493,25.6752026651745)) ;
#99380=CARTESIAN_POINT('Ctrl Pts',(38.630780914475,263.354595643023,25.6181202193676)) ;
#99381=CARTESIAN_POINT('Ctrl Pts',(38.611059726689,263.351689982552,25.5599425398626)) ;
#99382=CARTESIAN_POINT('Ctrl Pts',(38.5913424049923,263.3487848917,25.5017762653558)) ;
#99383=CARTESIAN_POINT('Ctrl Pts',(38.5748196579882,263.345879800847,25.4425156643958)) ;
#99384=CARTESIAN_POINT('Ctrl Pts',(38.5615972941645,263.342974709995,25.3825427625912)) ;
#99385=CARTESIAN_POINT('Ctrl Pts',(38.5483635797371,263.340067125297,25.3225183776586)) ;
#99386=CARTESIAN_POINT('Ctrl Pts',(38.5384360201161,263.337159540599,25.2617809668352)) ;
#99387=CARTESIAN_POINT('Ctrl Pts',(38.5318694613474,263.3342519559,25.2007237117402)) ;
#99388=CARTESIAN_POINT('Ctrl Pts',(38.5253002261765,263.331343186127,25.1396415708903)) ;
#99389=CARTESIAN_POINT('Ctrl Pts',(38.5220947511226,263.328434416354,25.0782398338323)) ;
#99390=CARTESIAN_POINT('Ctrl Pts',(38.5222557842831,263.32552564658,25.016914764314)) ;
#99391=CARTESIAN_POINT('Ctrl Pts',(38.5224171072803,263.322611641435,24.9554793183959)) ;
#99392=CARTESIAN_POINT('Ctrl Pts',(38.5259570180978,263.31969763629,24.8941213243164)) ;
#99393=CARTESIAN_POINT('Ctrl Pts',(38.532826150209,263.316783631145,24.8332341477001)) ;
#99394=CARTESIAN_POINT('Ctrl Pts',(38.5387202061188,263.31428327026,24.7809899314929)) ;
#99395=CARTESIAN_POINT('Ctrl Pts',(38.5470644947108,263.311782909374,24.7290924455471)) ;
#99396=CARTESIAN_POINT('Ctrl Pts',(38.5577980721274,263.309282548489,24.6777830230377)) ;
#99397=CARTESIAN_POINT('Ctrl Pts',(38.5704489428273,263.306335558773,24.6173084166072)) ;
#99398=CARTESIAN_POINT('Ctrl Pts',(38.5864685731215,263.303388569057,24.5574193685552)) ;
#99399=CARTESIAN_POINT('Ctrl Pts',(38.6057851883701,263.30044157934,24.4985161767056)) ;
#99400=CARTESIAN_POINT('Ctrl Pts',(38.6248974385109,263.297525768061,24.4402361663505)) ;
#99401=CARTESIAN_POINT('Ctrl Pts',(38.6472371113445,263.294609956782,24.382921750514)) ;
#99402=CARTESIAN_POINT('Ctrl Pts',(38.6726834954224,263.291694145503,24.3269505880656)) ;
#99403=CARTESIAN_POINT('Ctrl Pts',(38.6981058096377,263.288781092304,24.2710323690211)) ;
#99404=CARTESIAN_POINT('Ctrl Pts',(38.7266287987076,263.285868039106,24.2164553415877)) ;
#99405=CARTESIAN_POINT('Ctrl Pts',(38.7580830754285,263.282954985907,24.1635787477778)) ;
#99406=CARTESIAN_POINT('Ctrl Pts',(38.7895189214046,263.280043639622,24.1107331371952)) ;
#99407=CARTESIAN_POINT('Ctrl Pts',(38.8238823885485,263.277132293338,24.0595864165176)) ;
#99408=CARTESIAN_POINT('Ctrl Pts',(38.8609583578683,263.274220947053,24.0104729054478)) ;
#99409=CARTESIAN_POINT('Ctrl Pts',(38.8988090352623,263.27124876774,23.9603331600198)) ;
#99410=CARTESIAN_POINT('Ctrl Pts',(38.9394865908686,263.268276588428,23.912313033548)) ;
#99411=CARTESIAN_POINT('Ctrl Pts',(38.9827169258795,263.265304409115,23.8667351453348)) ;
#99412=CARTESIAN_POINT('Ctrl Pts',(39.0250778551607,263.262392003332,23.8220738745188)) ;
#99413=CARTESIAN_POINT('Ctrl Pts',(39.0698894207336,263.25947959755,23.7797578404798)) ;
#99414=CARTESIAN_POINT('Ctrl Pts',(39.1168561979467,263.256567191767,23.740053561592)) ;
#99415=CARTESIAN_POINT('Ctrl Pts',(39.1652688777606,263.253565125689,23.6991269608098)) ;
#99416=CARTESIAN_POINT('Ctrl Pts',(39.2159712282981,263.250563059612,23.6609759589132)) ;
#99417=CARTESIAN_POINT('Ctrl Pts',(39.2686048925834,263.247560993534,23.6258461530493)) ;
#99418=CARTESIAN_POINT('Ctrl Pts',(39.3212385568686,263.244558927457,23.5907163471854)) ;
#99419=CARTESIAN_POINT('Ctrl Pts',(39.375803011097,263.241556861379,23.5586079994299)) ;
#99420=CARTESIAN_POINT('Ctrl Pts',(39.4319120248721,263.238554795302,23.5297151930711)) ;
#99421=CARTESIAN_POINT('Ctrl Pts',(39.4328938139748,263.738513013137,23.5316344567886)) ;
#99422=CARTESIAN_POINT('Ctrl Pts',(39.7004812370594,263.724303920124,23.3946919530109)) ;
#99423=CARTESIAN_POINT('Ctrl Pts',(40.553309744137,263.684321281405,23.2013871196432)) ;
#99424=CARTESIAN_POINT('Ctrl Pts',(41.6546450483183,263.630047150456,23.8708672620324)) ;
#99425=CARTESIAN_POINT('Ctrl Pts',(41.8748774768301,263.58998211252,24.719421150606)) ;
#99426=CARTESIAN_POINT('Ctrl Pts',(41.8756052318586,263.575690620291,25.0217522355426)) ;
#99427=CARTESIAN_POINT('',(41.8792166192085,263.674309379709,25.0202225427276)) ;
#99428=CARTESIAN_POINT('Ctrl Pts',(39.4307622574477,263.837133669222,23.5274649509199)) ;
#99429=CARTESIAN_POINT('Ctrl Pts',(39.8937583329918,263.812379048163,23.2909189391529)) ;
#99430=CARTESIAN_POINT('Ctrl Pts',(41.0833957882848,263.761850881396,23.2773060297436)) ;
#99431=CARTESIAN_POINT('Ctrl Pts',(41.8396641814559,263.707576118226,24.3209713985087)) ;
#99432=CARTESIAN_POINT('Ctrl Pts',(41.879821877795,263.678055976114,24.9414011775634)) ;
#99433=CARTESIAN_POINT('Ctrl Pts',(41.8792166192085,263.674309379709,25.0202225427276)) ;
#99434=CARTESIAN_POINT('Ctrl Pts',(39.4319120248721,263.338461000729,23.5297151930711)) ;
#99435=CARTESIAN_POINT('Ctrl Pts',(39.4319044575765,263.338461403864,23.5297190897784)) ;
#99436=CARTESIAN_POINT('Ctrl Pts',(39.43189689031,263.338461806997,23.5297229865437)) ;
#99437=CARTESIAN_POINT('Ctrl Pts',(39.4058424989406,263.339849808694,23.5431399508344)) ;
#99438=CARTESIAN_POINT('Ctrl Pts',(39.3801506644007,263.341214537394,23.5572333935033)) ;
#99439=CARTESIAN_POINT('Ctrl Pts',(39.3160652980963,263.344615811434,23.5946040941535)) ;
#99440=CARTESIAN_POINT('Ctrl Pts',(39.2782120603637,263.346621717723,23.6187629767869)) ;
#99441=CARTESIAN_POINT('Ctrl Pts',(39.193782529487,263.351128734748,23.6775443528212)) ;
#99442=CARTESIAN_POINT('Ctrl Pts',(39.147942008179,263.353599803862,23.7131223859606)) ;
#99443=CARTESIAN_POINT('Ctrl Pts',(39.0200419202545,263.360736592239,23.8234681553043)) ;
#99444=CARTESIAN_POINT('Ctrl Pts',(38.9434506885163,263.36531733879,23.9040779328976)) ;
#99445=CARTESIAN_POINT('Ctrl Pts',(38.8611314484283,263.371363523247,24.0099771130338)) ;
#99446=CARTESIAN_POINT('Ctrl Pts',(38.8472647856884,263.372428427657,24.0286011092544)) ;
#99447=CARTESIAN_POINT('Ctrl Pts',(38.8243309000595,263.37428146348,24.0607761469446)) ;
#99448=CARTESIAN_POINT('Ctrl Pts',(38.8150670371125,263.375057781882,24.0741818732709)) ;
#99449=CARTESIAN_POINT('Ctrl Pts',(38.7935596389193,263.376928426921,24.1062955711805)) ;
#99450=CARTESIAN_POINT('Ctrl Pts',(38.781492816229,263.378032348686,24.1251160657035)) ;
#99451=CARTESIAN_POINT('Ctrl Pts',(38.7555884303837,263.380516773099,24.1673532300005)) ;
#99452=CARTESIAN_POINT('Ctrl Pts',(38.7419369548427,263.381905025912,24.1908766921485)) ;
#99453=CARTESIAN_POINT('Ctrl Pts',(38.6703601181564,263.389594067685,24.3214238146592)) ;
#99454=CARTESIAN_POINT('Ctrl Pts',(38.6236377447206,263.396147514065,24.4341764181685)) ;
#99455=CARTESIAN_POINT('Ctrl Pts',(38.5733502512279,263.405399704688,24.6063704400849)) ;
#99456=CARTESIAN_POINT('Ctrl Pts',(38.5600446374816,263.408312746396,24.6625444893242)) ;
#99457=CARTESIAN_POINT('Ctrl Pts',(38.5440720902454,263.412663317211,24.749822836433)) ;
#99458=CARTESIAN_POINT('Ctrl Pts',(38.5393333828028,263.414160205158,24.780499508075)) ;
#99459=CARTESIAN_POINT('Ctrl Pts',(38.5318059400181,263.417011639889,24.8401570440491)) ;
#99460=CARTESIAN_POINT('Ctrl Pts',(38.5289150858453,263.41836875821,24.8691136058087)) ;
#99461=CARTESIAN_POINT('Ctrl Pts',(38.5235849726333,263.421701726824,24.9415104177954)) ;
#99462=CARTESIAN_POINT('Ctrl Pts',(38.5220792577608,263.423649761571,24.9849984063511)) ;
#99463=CARTESIAN_POINT('Ctrl Pts',(38.5225011724418,263.427980741696,25.0836202657161)) ;
#99464=CARTESIAN_POINT('Ctrl Pts',(38.5254534333382,263.430337593687,25.1386991011082)) ;
#99465=CARTESIAN_POINT('Ctrl Pts',(38.5433683106536,263.437724376507,25.3123083204376)) ;
#99466=CARTESIAN_POINT('Ctrl Pts',(38.5682679108056,263.442628282687,25.4294228230056)) ;
#99467=CARTESIAN_POINT('Ctrl Pts',(38.6121239160881,263.449015500475,25.5635058129442)) ;
#99468=CARTESIAN_POINT('Ctrl Pts',(38.6192658359416,263.450014139772,25.5839880680574)) ;
#99469=CARTESIAN_POINT('Ctrl Pts',(38.6324676319988,263.451800418636,25.6196121796026)) ;
#99470=CARTESIAN_POINT('Ctrl Pts',(38.6383546152184,263.45257925519,25.6348140193688)) ;
#99471=CARTESIAN_POINT('Ctrl Pts',(38.6532696752001,263.454510667088,25.6717224767552)) ;
#99472=CARTESIAN_POINT('Ctrl Pts',(38.662533735973,263.455675059202,25.693328544745)) ;
#99473=CARTESIAN_POINT('Ctrl Pts',(38.6843174540834,263.458326602395,25.7413232974513)) ;
#99474=CARTESIAN_POINT('Ctrl Pts',(38.6970784603404,263.459823112037,25.7675941195224)) ;
#99475=CARTESIAN_POINT('Ctrl Pts',(38.7430329670758,263.464998175439,25.8562352314396)) ;
#99476=CARTESIAN_POINT('Ctrl Pts',(38.7794761933834,263.468751008503,25.9168356382739)) ;
#99477=CARTESIAN_POINT('Ctrl Pts',(38.8689869973971,263.47705043823,26.0464006856156)) ;
#99478=CARTESIAN_POINT('Ctrl Pts',(38.9238197952373,263.481565314494,26.1139098862064)) ;
#99479=CARTESIAN_POINT('Ctrl Pts',(39.0085115648262,263.487699226595,26.2030583254597)) ;
#99480=CARTESIAN_POINT('Ctrl Pts',(39.0342257126429,263.489469076468,26.2284325558702)) ;
#99481=CARTESIAN_POINT('Ctrl Pts',(39.0816018880483,263.492570921132,26.2722553214881)) ;
#99482=CARTESIAN_POINT('Ctrl Pts',(39.1029512817602,263.493915386886,26.2910198666659)) ;
#99483=CARTESIAN_POINT('Ctrl Pts',(39.1509963110643,263.496830437889,26.3311309188373)) ;
#99484=CARTESIAN_POINT('Ctrl Pts',(39.1778884361967,263.498390992979,26.3522225234828)) ;
#99485=CARTESIAN_POINT('Ctrl Pts',(39.2845272262057,263.504334138981,26.4307197364887)) ;
#99486=CARTESIAN_POINT('Ctrl Pts',(39.3686136710503,263.508496086443,26.481900875294)) ;
#99487=CARTESIAN_POINT('Ctrl Pts',(39.5429945408381,263.51669064325,26.568076525783)) ;
#99488=CARTESIAN_POINT('Ctrl Pts',(39.6327944658652,263.520713540441,26.6032134506906)) ;
#99489=CARTESIAN_POINT('Ctrl Pts',(39.747057515106,263.526089597176,26.6369354558312)) ;
#99490=CARTESIAN_POINT('Ctrl Pts',(39.7691422932421,263.527140559994,26.6429647667264)) ;
#99491=CARTESIAN_POINT('Ctrl Pts',(39.8071463279377,263.528979548858,26.6525090409327)) ;
#99492=CARTESIAN_POINT('Ctrl Pts',(39.8230053079206,263.529756410549,26.656247112356)) ;
#99493=CARTESIAN_POINT('Ctrl Pts',(39.8610600518077,263.531643721149,26.6646337367622)) ;
#99494=CARTESIAN_POINT('Ctrl Pts',(39.883298951415,263.532764376248,26.6690641204087)) ;
#99495=CARTESIAN_POINT('Ctrl Pts',(39.9329330077061,263.535294655861,26.6779102120752)) ;
#99496=CARTESIAN_POINT('Ctrl Pts',(39.9603617730635,263.536712456932,26.6820997311774)) ;
#99497=CARTESIAN_POINT('Ctrl Pts',(40.0509174967801,263.541431817705,26.693641383384)) ;
#99498=CARTESIAN_POINT('Ctrl Pts',(40.1143584020489,263.544797330329,26.6980875942634)) ;
#99499=CARTESIAN_POINT('Ctrl Pts',(40.2745680664189,263.553255944834,26.7001984256077)) ;
#99500=CARTESIAN_POINT('Ctrl Pts',(40.3711770065349,263.558309746368,26.6931139301979)) ;
#99501=CARTESIAN_POINT('Ctrl Pts',(40.5024958732422,263.564948060427,26.6719747306022)) ;
#99502=CARTESIAN_POINT('Ctrl Pts',(40.5381514245898,263.566728384874,26.6650409736292)) ;
#99503=CARTESIAN_POINT('Ctrl Pts',(40.6012675549001,263.569841170859,26.6506261536765)) ;
#99504=CARTESIAN_POINT('Ctrl Pts',(40.6288150989568,263.571186461844,26.6435936860961)) ;
#99505=CARTESIAN_POINT('Ctrl Pts',(40.6888966465598,263.574095343964,26.6266183050179)) ;
#99506=CARTESIAN_POINT('Ctrl Pts',(40.7213340270502,263.575649204437,26.6163791152147)) ;
#99507=CARTESIAN_POINT('Ctrl Pts',(40.846483191327,263.581602174001,26.5726484172548)) ;
#99508=CARTESIAN_POINT('Ctrl Pts',(40.9364855233383,263.585778126847,26.5319990247848)) ;
#99509=CARTESIAN_POINT('Ctrl Pts',(41.1065257039739,263.593996575398,26.4363720968552)) ;
#99510=CARTESIAN_POINT('Ctrl Pts',(41.1864047889597,263.598029362854,26.381894834373)) ;
#99511=CARTESIAN_POINT('Ctrl Pts',(41.2788632244251,263.603416216669,26.3063970321614)) ;
#99512=CARTESIAN_POINT('Ctrl Pts',(41.2962769625047,263.604466104081,26.2915741321219)) ;
#99513=CARTESIAN_POINT('Ctrl Pts',(41.3255691877186,263.606303890727,26.2655890022676)) ;
#99514=CARTESIAN_POINT('Ctrl Pts',(41.3375973185249,263.607080669057,26.2546016557788)) ;
#99515=CARTESIAN_POINT('Ctrl Pts',(41.3659919051207,263.608968672486,26.2278951511075)) ;
#99516=CARTESIAN_POINT('Ctrl Pts',(41.3822020408915,263.610090138224,26.212016835085)) ;
#99517=CARTESIAN_POINT('Ctrl Pts',(41.4175251398623,263.612622679174,26.175984281412)) ;
#99518=CARTESIAN_POINT('Ctrl Pts',(41.4364697245729,263.614041953369,26.1556742472572)) ;
#99519=CARTESIAN_POINT('Ctrl Pts',(41.4971640145001,263.618769609122,26.0872776849906)) ;
#99520=CARTESIAN_POINT('Ctrl Pts',(41.5366806976195,263.622142135583,26.0372848562047)) ;
#99521=CARTESIAN_POINT('Ctrl Pts',(41.6286871494578,263.630596959818,25.9061970663488)) ;
#99522=CARTESIAN_POINT('Ctrl Pts',(41.6772043377122,263.63563996828,25.8225846347282)) ;
#99523=CARTESIAN_POINT('Ctrl Pts',(41.7337212149292,263.64226861977,25.7023953005309)) ;
#99524=CARTESIAN_POINT('Ctrl Pts',(41.7481041164238,263.644049099289,25.6690376768099)) ;
#99525=CARTESIAN_POINT('Ctrl Pts',(41.7717946615636,263.647161987809,25.6087848524232)) ;
#99526=CARTESIAN_POINT('Ctrl Pts',(41.7815220283639,263.648507233998,25.5820709071693)) ;
#99527=CARTESIAN_POINT('Ctrl Pts',(41.8013840827117,263.651415824902,25.5228880041033)) ;
#99528=CARTESIAN_POINT('Ctrl Pts',(41.8112198767887,263.652969446806,25.4903318399547)) ;
#99529=CARTESIAN_POINT('Ctrl Pts',(41.8456271061157,263.658912480982,25.3625357860149)) ;
#99530=CARTESIAN_POINT('Ctrl Pts',(41.8627964239559,263.663079890315,25.2655053044538)) ;
#99531=CARTESIAN_POINT('Ctrl Pts',(41.8756534546012,263.669295346231,25.1185297823855)) ;
#99532=CARTESIAN_POINT('Ctrl Pts',(41.8777828183738,263.6713612837,25.0693691759817)) ;
#99533=CARTESIAN_POINT('Ctrl Pts',(41.877749617714,263.673464688334,25.0201877534197)) ;
#99534=CARTESIAN_POINT('Origin',(40.2,265.,25.0213203435596)) ;
#99535=CARTESIAN_POINT('',(41.0856881582581,263.,23.2689252008131)) ;
#99536=CARTESIAN_POINT('',(39.3481027319431,263.,23.2522518613699)) ;
#99537=CARTESIAN_POINT('Origin',(40.2,263.,25.0213203435596)) ;
#99538=CARTESIAN_POINT('',(42.1628844781328,263.339287097289,25.0223486673506)) ;
#99539=CARTESIAN_POINT('Ctrl Pts',(39.348102731943,263.,23.2522518613699)) ;
#99540=CARTESIAN_POINT('Ctrl Pts',(38.7751369603565,263.025773545707,23.5281642867049)) ;
#99541=CARTESIAN_POINT('Ctrl Pts',(37.9268112410175,263.077320637123,24.675932748524)) ;
#99542=CARTESIAN_POINT('Ctrl Pts',(38.6316894750799,263.154641274244,26.7065505405601)) ;
#99543=CARTESIAN_POINT('Ctrl Pts',(40.7072375606281,263.231961911367,27.2656011310219)) ;
#99544=CARTESIAN_POINT('Ctrl Pts',(42.0063554939681,263.293510420748,26.1536188564997)) ;
#99545=CARTESIAN_POINT('Ctrl Pts',(42.162562288311,263.329285384422,25.2698356603774)) ;
#99546=CARTESIAN_POINT('Ctrl Pts',(42.1613953394505,263.339286802389,25.0223551866513)) ;
#99547=CARTESIAN_POINT('',(42.1634995804015,263.839287219101,25.0200366912556)) ;
#99548=CARTESIAN_POINT('Ctrl Pts',(42.163499732132,263.33928721913,25.0223459738299)) ;
#99549=CARTESIAN_POINT('Ctrl Pts',(42.1635362473516,263.342109303692,24.9524400574562)) ;
#99550=CARTESIAN_POINT('Ctrl Pts',(42.1598351621169,263.344931388255,24.8825285938161)) ;
#99551=CARTESIAN_POINT('Ctrl Pts',(42.1524211029045,263.347753472817,24.813031873084)) ;
#99552=CARTESIAN_POINT('Ctrl Pts',(42.1450052456119,263.3505762418,24.7435182977953)) ;
#99553=CARTESIAN_POINT('Ctrl Pts',(42.1338746772063,263.353399010783,24.6744201360336)) ;
#99554=CARTESIAN_POINT('Ctrl Pts',(42.1191057347347,263.356221779765,24.6061511865783)) ;
#99555=CARTESIAN_POINT('Ctrl Pts',(42.1043178721143,263.359048164932,24.5377947793598)) ;
#99556=CARTESIAN_POINT('Ctrl Pts',(42.0858824313739,263.361874550098,24.4702701689134)) ;
#99557=CARTESIAN_POINT('Ctrl Pts',(42.0639264623263,263.364700935265,24.4039789525613)) ;
#99558=CARTESIAN_POINT('Ctrl Pts',(42.0419552698865,263.367529280134,24.3376417725266)) ;
#99559=CARTESIAN_POINT('Ctrl Pts',(42.0164588603084,263.370357625003,24.2725401310562)) ;
#99560=CARTESIAN_POINT('Ctrl Pts',(41.9876125998093,263.373185969872,24.2090559512568)) ;
#99561=CARTESIAN_POINT('Ctrl Pts',(41.9587122895671,263.376019614261,24.1454528200388)) ;
#99562=CARTESIAN_POINT('Ctrl Pts',(41.9264498115641,263.378853258649,24.0834736237973)) ;
#99563=CARTESIAN_POINT('Ctrl Pts',(41.8910464155505,263.381686903038,24.0234755307486)) ;
#99564=CARTESIAN_POINT('Ctrl Pts',(41.8705718281761,263.383325663896,23.9887772719162)) ;
#99565=CARTESIAN_POINT('Ctrl Pts',(41.8490475534782,263.384964424753,23.9547410743326)) ;
#99566=CARTESIAN_POINT('Ctrl Pts',(41.8265226751408,263.386603185611,23.9214311503893)) ;
#99567=CARTESIAN_POINT('Ctrl Pts',(41.7879759924163,263.389407586767,23.864428086906)) ;
#99568=CARTESIAN_POINT('Ctrl Pts',(41.7463588283396,263.392211987923,23.8093498190784)) ;
#99569=CARTESIAN_POINT('Ctrl Pts',(41.7018899125791,263.395016389079,23.7565441022848)) ;
#99570=CARTESIAN_POINT('Ctrl Pts',(41.6563626815685,263.397887532148,23.7024816628026)) ;
#99571=CARTESIAN_POINT('Ctrl Pts',(41.6078464321662,263.400758675217,23.6508018081332)) ;
#99572=CARTESIAN_POINT('Ctrl Pts',(41.5566234581295,263.403629818285,23.6018468345243)) ;
#99573=CARTESIAN_POINT('Ctrl Pts',(41.5067181249024,263.406427105134,23.5541511605222)) ;
#99574=CARTESIAN_POINT('Ctrl Pts',(41.4542440248292,263.409224391982,23.5090422217917)) ;
#99575=CARTESIAN_POINT('Ctrl Pts',(41.3995018974631,263.41202167883,23.4668019461186)) ;
#99576=CARTESIAN_POINT('Ctrl Pts',(41.3447906972838,263.414817385319,23.4245855345692)) ;
#99577=CARTESIAN_POINT('Ctrl Pts',(41.2878143977758,263.417613091809,23.3852348670235)) ;
#99578=CARTESIAN_POINT('Ctrl Pts',(41.2289072353883,263.420408798298,23.3489919813754)) ;
#99579=CARTESIAN_POINT('Ctrl Pts',(41.1700136034318,263.423203862639,23.3127574203833)) ;
#99580=CARTESIAN_POINT('Ctrl Pts',(41.1091904045308,263.42599892698,23.2796294785647)) ;
#99581=CARTESIAN_POINT('Ctrl Pts',(41.0467998285495,263.428793991322,23.2498062170654)) ;
#99582=CARTESIAN_POINT('Ctrl Pts',(40.9814533776778,263.431721477273,23.2185700205446)) ;
#99583=CARTESIAN_POINT('Ctrl Pts',(40.914387846715,263.434648963224,23.1909597090943)) ;
#99584=CARTESIAN_POINT('Ctrl Pts',(40.8460448913382,263.437576449175,23.1671471455072)) ;
#99585=CARTESIAN_POINT('Ctrl Pts',(40.7807177996198,263.440374749924,23.1443853916889)) ;
#99586=CARTESIAN_POINT('Ctrl Pts',(40.7142241584067,263.443173050673,23.1250933492162)) ;
#99587=CARTESIAN_POINT('Ctrl Pts',(40.6469648055212,263.445971351422,23.1093698440368)) ;
#99588=CARTESIAN_POINT('Ctrl Pts',(40.5796621742535,263.448771452752,23.0936362214859)) ;
#99589=CARTESIAN_POINT('Ctrl Pts',(40.5115933301378,263.451571554082,23.0814757916915)) ;
#99590=CARTESIAN_POINT('Ctrl Pts',(40.4431673895009,263.454371655413,23.0729359177639)) ;
#99591=CARTESIAN_POINT('Ctrl Pts',(40.3746364793251,263.457176052268,23.0643829431522)) ;
#99592=CARTESIAN_POINT('Ctrl Pts',(40.3057478649224,263.459980449123,23.0594616363704)) ;
#99593=CARTESIAN_POINT('Ctrl Pts',(40.2369127523885,263.462784845979,23.0581673442467)) ;
#99594=CARTESIAN_POINT('Ctrl Pts',(40.227593862907,263.463164504897,23.0579921231305)) ;
#99595=CARTESIAN_POINT('Ctrl Pts',(40.218275947807,263.463544163815,23.0578832989745)) ;
#99596=CARTESIAN_POINT('Ctrl Pts',(40.2089600200415,263.463923822733,23.0578407872512)) ;
#99597=CARTESIAN_POINT('Ctrl Pts',(40.1401422296188,263.466728405221,23.0575267484422)) ;
#99598=CARTESIAN_POINT('Ctrl Pts',(40.0711826945288,263.469532987708,23.0608344362365)) ;
#99599=CARTESIAN_POINT('Ctrl Pts',(40.0024920059422,263.472337570195,23.0677792402594)) ;
#99600=CARTESIAN_POINT('Ctrl Pts',(39.9321716504675,263.475208690598,23.0748888077662)) ;
#99601=CARTESIAN_POINT('Ctrl Pts',(39.8621335750225,263.478079811,23.0858103715288)) ;
#99602=CARTESIAN_POINT('Ctrl Pts',(39.7928195976218,263.480950931403,23.1005037542104)) ;
#99603=CARTESIAN_POINT('Ctrl Pts',(39.7252832136191,263.483748420413,23.1148203173669)) ;
#99604=CARTESIAN_POINT('Ctrl Pts',(39.6584347405197,263.486545909423,23.1327174457885)) ;
#99605=CARTESIAN_POINT('Ctrl Pts',(39.5926766314393,263.489343398433,23.1541056863763)) ;
#99606=CARTESIAN_POINT('Ctrl Pts',(39.5269555016547,263.492139314266,23.1754818992144)) ;
#99607=CARTESIAN_POINT('Ctrl Pts',(39.4623239815948,263.494935230098,23.2003451777175)) ;
#99608=CARTESIAN_POINT('Ctrl Pts',(39.399170461448,263.497731145931,23.2285559139195)) ;
#99609=CARTESIAN_POINT('Ctrl Pts',(39.33603129128,263.500526426465,23.2567602399728)) ;
#99610=CARTESIAN_POINT('Ctrl Pts',(39.2743698986226,263.503321706999,23.2883103140755)) ;
#99611=CARTESIAN_POINT('Ctrl Pts',(39.214554111061,263.506116987533,23.3230186477549)) ;
#99612=CARTESIAN_POINT('Ctrl Pts',(39.1519134864944,263.509044276893,23.3593661036352)) ;
#99613=CARTESIAN_POINT('Ctrl Pts',(39.0912976294582,263.511971566254,23.3991772600749)) ;
#99614=CARTESIAN_POINT('Ctrl Pts',(39.0330973689343,263.514898855614,23.4421843457393)) ;
#99615=CARTESIAN_POINT('Ctrl Pts',(38.9774570625523,263.517697387363,23.483299753152)) ;
#99616=CARTESIAN_POINT('Ctrl Pts',(38.9240246650862,263.520495919112,23.5273354697586)) ;
#99617=CARTESIAN_POINT('Ctrl Pts',(38.8731078398971,263.52329445086,23.5740161442092)) ;
#99618=CARTESIAN_POINT('Ctrl Pts',(38.8221581649257,263.526094788126,23.6207269354234)) ;
#99619=CARTESIAN_POINT('Ctrl Pts',(38.7737276331946,263.528895125391,23.6700857330352)) ;
#99620=CARTESIAN_POINT('Ctrl Pts',(38.7280860730949,263.531695462656,23.7217813323011)) ;
#99621=CARTESIAN_POINT('Ctrl Pts',(38.6823744142712,263.534500100827,23.7735563284048)) ;
#99622=CARTESIAN_POINT('Ctrl Pts',(38.6394605720532,263.537304738999,23.827674903296)) ;
#99623=CARTESIAN_POINT('Ctrl Pts',(38.5995725942992,263.54010937717,23.8837947969974)) ;
#99624=CARTESIAN_POINT('Ctrl Pts',(38.5941914898415,263.540487738065,23.8913656749201)) ;
#99625=CARTESIAN_POINT('Ctrl Pts',(38.5888653871444,263.54086609896,23.8989729372313)) ;
#99626=CARTESIAN_POINT('Ctrl Pts',(38.5835947824051,263.541244459855,23.9066157088999)) ;
#99627=CARTESIAN_POINT('Ctrl Pts',(38.544533355046,263.544048562487,23.9632577044803)) ;
#99628=CARTESIAN_POINT('Ctrl Pts',(38.5083813890949,263.546852665118,24.0220588127175)) ;
#99629=CARTESIAN_POINT('Ctrl Pts',(38.4753831864564,263.54965676775,24.082688841615)) ;
#99630=CARTESIAN_POINT('Ctrl Pts',(38.4415956242334,263.552527948134,24.1447692190344)) ;
#99631=CARTESIAN_POINT('Ctrl Pts',(38.4111150222394,263.555399128519,24.2087667739603)) ;
#99632=CARTESIAN_POINT('Ctrl Pts',(38.3841575439488,263.558270308903,24.2742939552694)) ;
#99633=CARTESIAN_POINT('Ctrl Pts',(38.357896670289,263.561067295495,24.3381278573537)) ;
#99634=CARTESIAN_POINT('Ctrl Pts',(38.3349792331306,263.563864282087,24.4034128045607)) ;
#99635=CARTESIAN_POINT('Ctrl Pts',(38.3155583761305,263.566661268679,24.4697661610644)) ;
#99636=CARTESIAN_POINT('Ctrl Pts',(38.2961484904738,263.569456675181,24.5360820328444)) ;
#99637=CARTESIAN_POINT('Ctrl Pts',(38.2802314017094,263.572252081683,24.6034646491454)) ;
#99638=CARTESIAN_POINT('Ctrl Pts',(38.2679109095461,263.575047488185,24.6715146881605)) ;
#99639=CARTESIAN_POINT('Ctrl Pts',(38.2555932439884,263.577842253356,24.7395491149247)) ;
#99640=CARTESIAN_POINT('Ctrl Pts',(38.2468706227258,263.580637018527,24.8082501807261)) ;
#99641=CARTESIAN_POINT('Ctrl Pts',(38.2417957115764,263.583431783699,24.8772085300274)) ;
#99642=CARTESIAN_POINT('Ctrl Pts',(38.2364792707681,263.586359559805,24.9494488060664)) ;
#99643=CARTESIAN_POINT('Ctrl Pts',(38.2351665055819,263.589287335912,25.0219708914576)) ;
#99644=CARTESIAN_POINT('Ctrl Pts',(38.2378567528721,263.592215112018,25.0943006679643)) ;
#99645=CARTESIAN_POINT('Ctrl Pts',(38.2404277594407,263.595013119335,25.1634245478339)) ;
#99646=CARTESIAN_POINT('Ctrl Pts',(38.2466543233326,263.597811126652,25.2323723027269)) ;
#99647=CARTESIAN_POINT('Ctrl Pts',(38.2564826038358,263.600609133968,25.3007346968185)) ;
#99648=CARTESIAN_POINT('Ctrl Pts',(38.2663172171149,263.603408944159,25.369141139686)) ;
#99649=CARTESIAN_POINT('Ctrl Pts',(38.2797580709152,263.60620875435,25.4369609933185)) ;
#99650=CARTESIAN_POINT('Ctrl Pts',(38.2967003789648,263.609008564541,25.5037960450898)) ;
#99651=CARTESIAN_POINT('Ctrl Pts',(38.3136687125046,263.611812675588,25.5707337638051)) ;
#99652=CARTESIAN_POINT('Ctrl Pts',(38.3341490833733,263.614616786635,25.6366831992214)) ;
#99653=CARTESIAN_POINT('Ctrl Pts',(38.3579874974153,263.617420897682,25.7012631281538)) ;
#99654=CARTESIAN_POINT('Ctrl Pts',(38.361229867408,263.617802297447,25.710046934968)) ;
#99655=CARTESIAN_POINT('Ctrl Pts',(38.3645342900422,263.618183697212,25.7188054404344)) ;
#99656=CARTESIAN_POINT('Ctrl Pts',(38.367900311567,263.618565096977,25.727537719191)) ;
#99657=CARTESIAN_POINT('Ctrl Pts',(38.3926496156565,263.621369410229,25.791743435272)) ;
#99658=CARTESIAN_POINT('Ctrl Pts',(38.4208232163479,263.62417372348,25.8547637149043)) ;
#99659=CARTESIAN_POINT('Ctrl Pts',(38.4522861380892,263.626978036731,25.9162105641369)) ;
#99660=CARTESIAN_POINT('Ctrl Pts',(38.4844989785645,263.629849190788,25.9791219990097)) ;
#99661=CARTESIAN_POINT('Ctrl Pts',(38.5201598569172,263.632720344845,26.040383521597)) ;
#99662=CARTESIAN_POINT('Ctrl Pts',(38.5590706117971,263.635591498902,26.0995981338029)) ;
#99663=CARTESIAN_POINT('Ctrl Pts',(38.5969791725281,263.63838870287,26.1572876011469)) ;
#99664=CARTESIAN_POINT('Ctrl Pts',(38.6379719273339,263.641185906837,26.2130338976945)) ;
#99665=CARTESIAN_POINT('Ctrl Pts',(38.6818191935624,263.643983110805,26.2664947445832)) ;
#99666=CARTESIAN_POINT('Ctrl Pts',(38.7256417206521,263.646778736558,26.3199254282388)) ;
#99667=CARTESIAN_POINT('Ctrl Pts',(38.7723152545264,263.649574362311,26.3710728450201)) ;
#99668=CARTESIAN_POINT('Ctrl Pts',(38.8215685088218,263.652369988063,26.4196260591055)) ;
#99669=CARTESIAN_POINT('Ctrl Pts',(38.870810490521,263.655164973981,26.4681681608129)) ;
#99670=CARTESIAN_POINT('Ctrl Pts',(38.922630672812,263.657959959898,26.5141168972352)) ;
#99671=CARTESIAN_POINT('Ctrl Pts',(38.9767206494171,263.660754945816,26.5571979039261)) ;
#99672=CARTESIAN_POINT('Ctrl Pts',(39.0333763766254,263.663682511506,26.602322452246)) ;
#99673=CARTESIAN_POINT('Ctrl Pts',(39.0925221659636,263.666610077197,26.6443000437003)) ;
#99674=CARTESIAN_POINT('Ctrl Pts',(39.1537662292884,263.669537642887,26.6828639472675)) ;
#99675=CARTESIAN_POINT('Ctrl Pts',(39.21230460047,263.672335872099,26.7197241420141)) ;
#99676=CARTESIAN_POINT('Ctrl Pts',(39.2727592794513,263.67513410131,26.7534657211203)) ;
#99677=CARTESIAN_POINT('Ctrl Pts',(39.3347619023668,263.677932330522,26.783902337228)) ;
#99678=CARTESIAN_POINT('Ctrl Pts',(39.3968044771535,263.680732362794,26.8143585654055)) ;
#99679=CARTESIAN_POINT('Ctrl Pts',(39.4603965330109,263.683532395067,26.8415054011816)) ;
#99680=CARTESIAN_POINT('Ctrl Pts',(39.5251500779897,263.686332427339,26.865204784831)) ;
#99681=CARTESIAN_POINT('Ctrl Pts',(39.5900030547217,263.689136759177,26.8889405598666)) ;
#99682=CARTESIAN_POINT('Ctrl Pts',(39.6560206129491,263.691941091015,26.9092181821856)) ;
#99683=CARTESIAN_POINT('Ctrl Pts',(39.7228010388372,263.694745422853,26.9259498092209)) ;
#99684=CARTESIAN_POINT('Ctrl Pts',(39.7318525675763,263.695125526602,26.9282176414629)) ;
#99685=CARTESIAN_POINT('Ctrl Pts',(39.740918099865,263.695505630351,26.9304204058221)) ;
#99686=CARTESIAN_POINT('Ctrl Pts',(39.7499966261111,263.695885734099,26.9325579565969)) ;
#99687=CARTESIAN_POINT('Ctrl Pts',(39.8169755789748,263.698690038497,26.9483282378862)) ;
#99688=CARTESIAN_POINT('Ctrl Pts',(39.8849066936081,263.701494342894,26.9606021865827)) ;
#99689=CARTESIAN_POINT('Ctrl Pts',(39.9533934422283,263.704298647291,26.9692724619814)) ;
#99690=CARTESIAN_POINT('Ctrl Pts',(40.0235128209001,263.707169802455,26.9781494248409)) ;
#99691=CARTESIAN_POINT('Ctrl Pts',(40.0942141853674,263.710040957619,26.9832484865268)) ;
#99692=CARTESIAN_POINT('Ctrl Pts',(40.1650579347143,263.712912112783,26.9845094078307)) ;
#99693=CARTESIAN_POINT('Ctrl Pts',(40.2340767988411,263.715709309006,26.9857378486875)) ;
#99694=CARTESIAN_POINT('Ctrl Pts',(40.3032302807727,263.71850650523,26.983323498587)) ;
#99695=CARTESIAN_POINT('Ctrl Pts',(40.3721061957367,263.721303701453,26.9772630082073)) ;
#99696=CARTESIAN_POINT('Ctrl Pts',(40.4409432607295,263.724099319898,26.9712059362922)) ;
#99697=CARTESIAN_POINT('Ctrl Pts',(40.5095025848152,263.726894938342,26.9615068481037)) ;
#99698=CARTESIAN_POINT('Ctrl Pts',(40.5773744049012,263.729690556786,26.9482144269294)) ;
#99699=CARTESIAN_POINT('Ctrl Pts',(40.6452307020316,263.732485535845,26.934925045863)) ;
#99700=CARTESIAN_POINT('Ctrl Pts',(40.7123993293839,263.735280514903,26.9180440580058)) ;
#99701=CARTESIAN_POINT('Ctrl Pts',(40.7784797918224,263.738075493962,26.8976714249016)) ;
#99702=CARTESIAN_POINT('Ctrl Pts',(40.8476951170664,263.741003067067,26.8763323123356)) ;
#99703=CARTESIAN_POINT('Ctrl Pts',(40.9157158954227,263.743930640172,26.8511621496684)) ;
#99704=CARTESIAN_POINT('Ctrl Pts',(40.9821009073791,263.746858213277,26.8223340638507)) ;
#99705=CARTESIAN_POINT('Ctrl Pts',(41.0455528173557,263.749656436846,26.7947796949925)) ;
#99706=CARTESIAN_POINT('Ctrl Pts',(41.1075100309649,263.752454660415,26.7638841087761)) ;
#99707=CARTESIAN_POINT('Ctrl Pts',(41.1676109269251,263.755252883985,26.7298464171374)) ;
#99708=CARTESIAN_POINT('Ctrl Pts',(41.2277505586288,263.758052911043,26.6957867878009)) ;
#99709=CARTESIAN_POINT('Ctrl Pts',(41.2860310811265,263.7608529381,26.6585812847864)) ;
#99710=CARTESIAN_POINT('Ctrl Pts',(41.3421196810525,263.763652965158,26.6184724603451)) ;
#99711=CARTESIAN_POINT('Ctrl Pts',(41.3982944203982,263.766457292425,26.5783020378097)) ;
#99712=CARTESIAN_POINT('Ctrl Pts',(41.4522701434347,263.769261619692,26.5352197043128)) ;
#99713=CARTESIAN_POINT('Ctrl Pts',(41.5037477688255,263.772065946958,26.489507663108)) ;
#99714=CARTESIAN_POINT('Ctrl Pts',(41.5107258337244,263.772446088379,26.483311153697)) ;
#99715=CARTESIAN_POINT('Ctrl Pts',(41.5176580530097,263.7728262298,26.4770663759933)) ;
#99716=CARTESIAN_POINT('Ctrl Pts',(41.5245437368096,263.773206371221,26.4707740817929)) ;
#99717=CARTESIAN_POINT('Ctrl Pts',(41.57461281309,263.775970559987,26.4250198230361)) ;
#99718=CARTESIAN_POINT('Ctrl Pts',(41.6224125805603,263.778734748753,26.3765726870436)) ;
#99719=CARTESIAN_POINT('Ctrl Pts',(41.6676353975584,263.781498937519,26.3256893825335)) ;
#99720=CARTESIAN_POINT('Ctrl Pts',(41.712801126539,263.78425963685,26.2748703116817)) ;
#99721=CARTESIAN_POINT('Ctrl Pts',(41.7553960200713,263.787020336182,26.2216215386591)) ;
#99722=CARTESIAN_POINT('Ctrl Pts',(41.7951474334239,263.789781035513,26.1662382077058)) ;
#99723=CARTESIAN_POINT('Ctrl Pts',(41.8348629859507,263.792539244343,26.1109048395543)) ;
#99724=CARTESIAN_POINT('Ctrl Pts',(41.8717398514875,263.795297453173,26.053441137395)) ;
#99725=CARTESIAN_POINT('Ctrl Pts',(41.9055453353879,263.798055662003,25.9941756046013)) ;
#99726=CARTESIAN_POINT('Ctrl Pts',(41.9393324965953,263.800812375874,25.9349421939379)) ;
#99727=CARTESIAN_POINT('Ctrl Pts',(41.9700513297317,263.803569089744,25.8739093259822)) ;
#99728=CARTESIAN_POINT('Ctrl Pts',(41.997513287225,263.806325803615,25.8114331407283)) ;
#99729=CARTESIAN_POINT('Ctrl Pts',(42.0249844738963,263.809083443939,25.7489359590164)) ;
#99730=CARTESIAN_POINT('Ctrl Pts',(42.0491963823633,263.811841084262,25.6849949460299)) ;
#99731=CARTESIAN_POINT('Ctrl Pts',(42.0700077617375,263.814598724586,25.6199882156234)) ;
#99732=CARTESIAN_POINT('Ctrl Pts',(42.0908213077346,263.817356652001,25.554974717522)) ;
#99733=CARTESIAN_POINT('Ctrl Pts',(42.1082334793487,263.820114579415,25.4888957648959)) ;
#99734=CARTESIAN_POINT('Ctrl Pts',(42.122153100212,263.82287250683,25.4221441319574)) ;
#99735=CARTESIAN_POINT('Ctrl Pts',(42.1360919737274,263.825634248818,25.3553001727996)) ;
#99736=CARTESIAN_POINT('Ctrl Pts',(42.1465285576744,263.828395990807,25.2877821713475)) ;
#99737=CARTESIAN_POINT('Ctrl Pts',(42.1534231331806,263.831157732795,25.2199917122938)) ;
#99738=CARTESIAN_POINT('Ctrl Pts',(42.1601881094651,263.833867561564,25.1534755290423)) ;
#99739=CARTESIAN_POINT('Ctrl Pts',(42.1635431603993,263.836577390332,25.0866975052807)) ;
#99740=CARTESIAN_POINT('Ctrl Pts',(42.1634995804015,263.839287219101,25.0200366912556)) ;
#99741=CARTESIAN_POINT('',(42.1634995162458,264.339287219108,25.0226986405015)) ;
#99742=CARTESIAN_POINT('Ctrl Pts',(42.163499580401,263.83928721913,25.0200366905463)) ;
#99743=CARTESIAN_POINT('Ctrl Pts',(42.1634393268694,263.843033815535,24.9278717652068)) ;
#99744=CARTESIAN_POINT('Ctrl Pts',(42.1568885505834,263.846780411939,24.8359264198449)) ;
#99745=CARTESIAN_POINT('Ctrl Pts',(42.1439469198114,263.850527008343,24.7449100996181)) ;
#99746=CARTESIAN_POINT('Ctrl Pts',(42.1342602498124,263.853331295038,24.6767853729825)) ;
#99747=CARTESIAN_POINT('Ctrl Pts',(42.1209705345478,263.856135581733,24.609046166368)) ;
#99748=CARTESIAN_POINT('Ctrl Pts',(42.1041220948803,263.858939868429,24.5421008763124)) ;
#99749=CARTESIAN_POINT('Ctrl Pts',(42.0868718893598,263.861811025805,24.4735592169732)) ;
#99750=CARTESIAN_POINT('Ctrl Pts',(42.0658910379676,263.864682183181,24.405850346248)) ;
#99751=CARTESIAN_POINT('Ctrl Pts',(42.0412834107829,263.867553340558,24.339405648619)) ;
#99752=CARTESIAN_POINT('Ctrl Pts',(42.0173098391839,263.870350517889,24.2746730068238)) ;
#99753=CARTESIAN_POINT('Ctrl Pts',(41.9898943245674,263.87314769522,24.2111406620449)) ;
#99754=CARTESIAN_POINT('Ctrl Pts',(41.9591837468858,263.875944872551,24.1491937502872)) ;
#99755=CARTESIAN_POINT('Ctrl Pts',(41.9284904961072,263.878740471716,24.0872817889672)) ;
#99756=CARTESIAN_POINT('Ctrl Pts',(41.8945060876673,263.88153607088,24.0269539214354)) ;
#99757=CARTESIAN_POINT('Ctrl Pts',(41.8574249850417,263.884331670045,23.9685740925762)) ;
#99758=CARTESIAN_POINT('Ctrl Pts',(41.8203523679988,263.887126629468,23.9102076232677)) ;
#99759=CARTESIAN_POINT('Ctrl Pts',(41.7801847257056,263.889921588892,23.8537887183574)) ;
#99760=CARTESIAN_POINT('Ctrl Pts',(41.7371609110175,263.892716548316,23.7996540292005)) ;
#99761=CARTESIAN_POINT('Ctrl Pts',(41.6920954442125,263.895644139745,23.7429504324857)) ;
#99762=CARTESIAN_POINT('Ctrl Pts',(41.6438963087687,263.898571731175,23.6887537205247)) ;
#99763=CARTESIAN_POINT('Ctrl Pts',(41.5928853393019,263.901499322604,23.6374118633638)) ;
#99764=CARTESIAN_POINT('Ctrl Pts',(41.5441288563539,263.904297525875,23.5883391166714)) ;
#99765=CARTESIAN_POINT('Ctrl Pts',(41.4928042619471,263.907095729145,23.541874496461)) ;
#99766=CARTESIAN_POINT('Ctrl Pts',(41.4392286140248,263.909893932416,23.4982823623582)) ;
#99767=CARTESIAN_POINT('Ctrl Pts',(41.3856184397523,263.912693938964,23.4546621356919)) ;
#99768=CARTESIAN_POINT('Ctrl Pts',(41.3297547183872,263.915493945512,23.413918366189)) ;
#99769=CARTESIAN_POINT('Ctrl Pts',(41.2719844854997,263.91829395206,23.3762727719533)) ;
#99770=CARTESIAN_POINT('Ctrl Pts',(41.2141255331622,263.92109825866,23.3385693642685)) ;
#99771=CARTESIAN_POINT('Ctrl Pts',(41.1543546506205,263.92390256526,23.3039738647254)) ;
#99772=CARTESIAN_POINT('Ctrl Pts',(41.0930435295117,263.926706871861,23.2726621424244)) ;
#99773=CARTESIAN_POINT('Ctrl Pts',(41.0847298749895,263.92708712973,23.2684163410593)) ;
#99774=CARTESIAN_POINT('Ctrl Pts',(41.0763879291037,263.927467387599,23.2642308447549)) ;
#99775=CARTESIAN_POINT('Ctrl Pts',(41.0680186440471,263.927847645467,23.2601060228176)) ;
#99776=CARTESIAN_POINT('Ctrl Pts',(41.0062977660224,263.930651929153,23.2296867420853)) ;
#99777=CARTESIAN_POINT('Ctrl Pts',(40.9428633334637,263.933456212838,23.2024603023848)) ;
#99778=CARTESIAN_POINT('Ctrl Pts',(40.8780775986114,263.936260496523,23.1786204167507)) ;
#99779=CARTESIAN_POINT('Ctrl Pts',(40.8117469110722,263.939131654276,23.1542120186896)) ;
#99780=CARTESIAN_POINT('Ctrl Pts',(40.744000064422,263.942002812029,23.1333540793622)) ;
#99781=CARTESIAN_POINT('Ctrl Pts',(40.675251878674,263.944873969781,23.1162040999102)) ;
#99782=CARTESIAN_POINT('Ctrl Pts',(40.6082751827735,263.947671144101,23.0994960377853)) ;
#99783=CARTESIAN_POINT('Ctrl Pts',(40.5403486362851,263.950468318421,23.0863072672656)) ;
#99784=CARTESIAN_POINT('Ctrl Pts',(40.4718731205651,263.95326549274,23.0767336891998)) ;
#99785=CARTESIAN_POINT('Ctrl Pts',(40.4034362385558,263.956061088901,23.0671655125223)) ;
#99786=CARTESIAN_POINT('Ctrl Pts',(40.3344514837967,263.958856685062,23.0612085479421)) ;
#99787=CARTESIAN_POINT('Ctrl Pts',(40.2653290723423,263.961652281223,23.0589074506375)) ;
#99788=CARTESIAN_POINT('Ctrl Pts',(40.1962224784314,263.964447237657,23.0566068799017)) ;
#99789=CARTESIAN_POINT('Ctrl Pts',(40.1269787773539,263.967242194091,23.0579605307881)) ;
#99790=CARTESIAN_POINT('Ctrl Pts',(40.058010679081,263.970037150525,23.0629610091307)) ;
#99791=CARTESIAN_POINT('Ctrl Pts',(39.9857696195808,263.972964744863,23.0681987909823)) ;
#99792=CARTESIAN_POINT('Ctrl Pts',(39.9138315536871,263.975892339202,23.0774381490376)) ;
#99793=CARTESIAN_POINT('Ctrl Pts',(39.8426653384802,263.97881993354,23.0906095444816)) ;
#99794=CARTESIAN_POINT('Ctrl Pts',(39.7746445318474,263.981618133892,23.1031987898134)) ;
#99795=CARTESIAN_POINT('Ctrl Pts',(39.7073292681962,263.984416334243,23.1193796467941)) ;
#99796=CARTESIAN_POINT('Ctrl Pts',(39.6411166615528,263.987214534595,23.1390393698455)) ;
#99797=CARTESIAN_POINT('Ctrl Pts',(39.5748613840908,263.990014538251,23.1587117626364)) ;
#99798=CARTESIAN_POINT('Ctrl Pts',(39.5097106367583,263.992814541907,23.1818673202465)) ;
#99799=CARTESIAN_POINT('Ctrl Pts',(39.4460432254316,263.995614545563,23.2083444937253)) ;
#99800=CARTESIAN_POINT('Ctrl Pts',(39.3822780367358,263.998418849331,23.2348623295824)) ;
#99801=CARTESIAN_POINT('Ctrl Pts',(39.3200011657801,264.001223153099,23.2647117450625)) ;
#99802=CARTESIAN_POINT('Ctrl Pts',(39.2595674604394,264.004027456867,23.2976849736117)) ;
#99803=CARTESIAN_POINT('Ctrl Pts',(39.2513723989487,264.004407732107,23.3021562803764)) ;
#99804=CARTESIAN_POINT('Ctrl Pts',(39.2432111863563,264.004788007347,23.3066849645074)) ;
#99805=CARTESIAN_POINT('Ctrl Pts',(39.2350846647403,264.005168282588,23.3112704478604)) ;
#99806=CARTESIAN_POINT('Ctrl Pts',(39.1751568842898,264.007972563704,23.3450853877112)) ;
#99807=CARTESIAN_POINT('Ctrl Pts',(39.1168994297693,264.01077684482,23.3821159857374)) ;
#99808=CARTESIAN_POINT('Ctrl Pts',(39.0606765621799,264.013581125937,23.4221723347644)) ;
#99809=CARTESIAN_POINT('Ctrl Pts',(39.0031128823909,264.01645228401,23.4631839541955)) ;
#99810=CARTESIAN_POINT('Ctrl Pts',(38.9476825722119,264.019323442084,23.5073673238714)) ;
#99811=CARTESIAN_POINT('Ctrl Pts',(38.8947496350886,264.022194600158,23.5544687031752)) ;
#99812=CARTESIAN_POINT('Ctrl Pts',(38.8431807197224,264.024991771745,23.600356333353)) ;
#99813=CARTESIAN_POINT('Ctrl Pts',(38.7939824046442,264.027788943331,23.6490130484392)) ;
#99814=CARTESIAN_POINT('Ctrl Pts',(38.7474599613417,264.030586114918,23.7001618799019)) ;
#99815=CARTESIAN_POINT('Ctrl Pts',(38.7009637667907,264.033381708293,23.7512818523263)) ;
#99816=CARTESIAN_POINT('Ctrl Pts',(38.6571407752526,264.036177301668,23.804890790839)) ;
#99817=CARTESIAN_POINT('Ctrl Pts',(38.6162592032904,264.038972895043,23.8606751183345)) ;
#99818=CARTESIAN_POINT('Ctrl Pts',(38.5753869871292,264.041767848643,23.9164466795142)) ;
#99819=CARTESIAN_POINT('Ctrl Pts',(38.5374551413506,264.044562802242,23.974392247734)) ;
#99820=CARTESIAN_POINT('Ctrl Pts',(38.5026903060573,264.047357755842,24.0341668332846)) ;
#99821=CARTESIAN_POINT('Ctrl Pts',(38.4662755952239,264.050285352831,24.09677821141)) ;
#99822=CARTESIAN_POINT('Ctrl Pts',(38.4333363101176,264.05321294982,24.1613960540302)) ;
#99823=CARTESIAN_POINT('Ctrl Pts',(38.4040794362206,264.056140546809,24.22759395582)) ;
#99824=CARTESIAN_POINT('Ctrl Pts',(38.3761157138824,264.058938744238,24.2908659154811)) ;
#99825=CARTESIAN_POINT('Ctrl Pts',(38.3515158675236,264.061736941667,24.3555807041219)) ;
#99826=CARTESIAN_POINT('Ctrl Pts',(38.3304107415181,264.064535139096,24.4213467986687)) ;
#99827=CARTESIAN_POINT('Ctrl Pts',(38.3092920144767,264.067335139802,24.4871552756684)) ;
#99828=CARTESIAN_POINT('Ctrl Pts',(38.2916726140117,264.070135140508,24.5540159359703)) ;
#99829=CARTESIAN_POINT('Ctrl Pts',(38.2776327573044,264.072935141214,24.6215248530763)) ;
#99830=CARTESIAN_POINT('Ctrl Pts',(38.2635713389277,264.075739442012,24.6891374468065)) ;
#99831=CARTESIAN_POINT('Ctrl Pts',(38.2531005018651,264.078543742811,24.7573998023813)) ;
#99832=CARTESIAN_POINT('Ctrl Pts',(38.2462487852448,264.08134804361,24.8259017138375)) ;
#99833=CARTESIAN_POINT('Ctrl Pts',(38.2453196219938,264.081728335644,24.8351912776466)) ;
#99834=CARTESIAN_POINT('Ctrl Pts',(38.2444569364807,264.082108627677,24.8444852468057)) ;
#99835=CARTESIAN_POINT('Ctrl Pts',(38.2436607261533,264.082488919711,24.8537825997379)) ;
#99836=CARTESIAN_POINT('Ctrl Pts',(38.2377894554891,264.085293200669,24.9223414637035)) ;
#99837=CARTESIAN_POINT('Ctrl Pts',(38.2355156869784,264.088097481628,24.991334410235)) ;
#99838=CARTESIAN_POINT('Ctrl Pts',(38.2368880163663,264.090901762587,25.060353530899)) ;
#99839=CARTESIAN_POINT('Ctrl Pts',(38.2382930733799,264.093772920681,25.1310186353642)) ;
#99840=CARTESIAN_POINT('Ctrl Pts',(38.2435205047617,264.096644078774,25.2017106737457)) ;
#99841=CARTESIAN_POINT('Ctrl Pts',(38.2525660465842,264.099515236868,25.271985951658)) ;
#99842=CARTESIAN_POINT('Ctrl Pts',(38.2613784947858,264.102312408389,25.3404503132856)) ;
#99843=CARTESIAN_POINT('Ctrl Pts',(38.2738145764158,264.10510957991,25.4085186194253)) ;
#99844=CARTESIAN_POINT('Ctrl Pts',(38.2898177240288,264.107906751431,25.4757825780363)) ;
#99845=CARTESIAN_POINT('Ctrl Pts',(38.3058118425898,264.110702344774,25.5430085860018)) ;
#99846=CARTESIAN_POINT('Ctrl Pts',(38.3253689206372,264.113497938118,25.6094306737226)) ;
#99847=CARTESIAN_POINT('Ctrl Pts',(38.3483812619677,264.116293531461,25.6746505043264)) ;
#99848=CARTESIAN_POINT('Ctrl Pts',(38.3713883371747,264.119088485064,25.7398554100829)) ;
#99849=CARTESIAN_POINT('Ctrl Pts',(38.397848942836,264.121883438666,25.8038581457887)) ;
#99850=CARTESIAN_POINT('Ctrl Pts',(38.4276059949864,264.124678392269,25.8662769939221)) ;
#99851=CARTESIAN_POINT('Ctrl Pts',(38.4587752630291,264.127605989316,25.9316581277304)) ;
#99852=CARTESIAN_POINT('Ctrl Pts',(38.4935614451515,264.130533586363,25.9953007515779)) ;
#99853=CARTESIAN_POINT('Ctrl Pts',(38.5317291392618,264.13346118341,26.0567934649934)) ;
#99854=CARTESIAN_POINT('Ctrl Pts',(38.5682098246742,264.136259380927,26.1155682059243)) ;
#99855=CARTESIAN_POINT('Ctrl Pts',(38.6077790592181,264.139057578443,26.1723786961002)) ;
#99856=CARTESIAN_POINT('Ctrl Pts',(38.6501873075505,264.14185577596,26.2268960849888)) ;
#99857=CARTESIAN_POINT('Ctrl Pts',(38.6926228859955,264.144655776783,26.2814486077589)) ;
#99858=CARTESIAN_POINT('Ctrl Pts',(38.7379008005125,264.147455777606,26.333704720125)) ;
#99859=CARTESIAN_POINT('Ctrl Pts',(38.7857327218907,264.150255778429,26.3833703852502)) ;
#99860=CARTESIAN_POINT('Ctrl Pts',(38.8336381016924,264.153060079386,26.4331123249919)) ;
#99861=CARTESIAN_POINT('Ctrl Pts',(38.8841049558928,264.155864380342,26.4802555512367)) ;
#99862=CARTESIAN_POINT('Ctrl Pts',(38.9368106260223,264.158668681298,26.5245451622311)) ;
#99863=CARTESIAN_POINT('Ctrl Pts',(38.9439580530727,264.159048973143,26.5305512857258)) ;
#99864=CARTESIAN_POINT('Ctrl Pts',(38.9511466079102,264.159429264988,26.5365049955676)) ;
#99865=CARTESIAN_POINT('Ctrl Pts',(38.9583754454666,264.159809556832,26.5424057177512)) ;
#99866=CARTESIAN_POINT('Ctrl Pts',(39.0116811190239,264.162613840753,26.5859178271355)) ;
#99867=CARTESIAN_POINT('Ctrl Pts',(39.067374064098,264.165418124673,26.6267038710569)) ;
#99868=CARTESIAN_POINT('Ctrl Pts',(39.1251448299156,264.168222408594,26.6644936799252)) ;
#99869=CARTESIAN_POINT('Ctrl Pts',(39.1842932560943,264.171093566317,26.70318466296)) ;
#99870=CARTESIAN_POINT('Ctrl Pts',(39.2456195358669,264.173964724041,26.7387342754357)) ;
#99871=CARTESIAN_POINT('Ctrl Pts',(39.3087548572949,264.176835881764,26.7708958193836)) ;
#99872=CARTESIAN_POINT('Ctrl Pts',(39.3702633228545,264.179633056182,26.802228632356)) ;
#99873=CARTESIAN_POINT('Ctrl Pts',(39.4334882579985,264.182430230599,26.8303456470777)) ;
#99874=CARTESIAN_POINT('Ctrl Pts',(39.4980605888599,264.185227405017,26.855063322575)) ;
#99875=CARTESIAN_POINT('Ctrl Pts',(39.5625964869995,264.188023001225,26.8797670519722)) ;
#99876=CARTESIAN_POINT('Ctrl Pts',(39.6284778178391,264.190818597432,26.9010750743839)) ;
#99877=CARTESIAN_POINT('Ctrl Pts',(39.6953148947306,264.19361419364,26.91885168573)) ;
#99878=CARTESIAN_POINT('Ctrl Pts',(39.762136675821,264.19640915007,26.9366242288625)) ;
#99879=CARTESIAN_POINT('Ctrl Pts',(39.8299132976171,264.1992041065,26.9508668411143)) ;
#99880=CARTESIAN_POINT('Ctrl Pts',(39.898240945861,264.20199906293,26.9614939758011)) ;
#99881=CARTESIAN_POINT('Ctrl Pts',(39.9698111600169,264.204926657182,26.9726254331971)) ;
#99882=CARTESIAN_POINT('Ctrl Pts',(40.0419854358326,264.207854251434,26.9797895834628)) ;
#99883=CARTESIAN_POINT('Ctrl Pts',(40.1142912819507,264.210781845686,26.982948816449)) ;
#99884=CARTESIAN_POINT('Ctrl Pts',(40.1834013488205,264.213580045906,26.985968417417)) ;
#99885=CARTESIAN_POINT('Ctrl Pts',(40.2526310910439,264.216378246127,26.9853297205025)) ;
#99886=CARTESIAN_POINT('Ctrl Pts',(40.3215682148443,264.219176446347,26.9810533404598)) ;
#99887=CARTESIAN_POINT('Ctrl Pts',(40.3905497642044,264.221976449828,26.9767742045642)) ;
#99888=CARTESIAN_POINT('Ctrl Pts',(40.4592378360349,264.224776453309,26.9688527759086)) ;
#99889=CARTESIAN_POINT('Ctrl Pts',(40.5272270083716,264.22757645679,26.957361338733)) ;
#99890=CARTESIAN_POINT('Ctrl Pts',(40.5953205937682,264.230380760322,26.9458522538045)) ;
#99891=CARTESIAN_POINT('Ctrl Pts',(40.6627126646325,264.233185063854,26.93076233205)) ;
#99892=CARTESIAN_POINT('Ctrl Pts',(40.7290107572647,264.235989367386,26.9122142773111)) ;
#99893=CARTESIAN_POINT('Ctrl Pts',(40.7380010614685,264.236369642909,26.9096990819583)) ;
#99894=CARTESIAN_POINT('Ctrl Pts',(40.7469712774647,264.236749918432,26.9071203697556)) ;
#99895=CARTESIAN_POINT('Ctrl Pts',(40.7559204547825,264.237130193955,26.9044785148119)) ;
#99896=CARTESIAN_POINT('Ctrl Pts',(40.8219148662837,264.2399344807,26.8849965383031)) ;
#99897=CARTESIAN_POINT('Ctrl Pts',(40.8870043490843,264.242738767445,26.8620057637231)) ;
#99898=CARTESIAN_POINT('Ctrl Pts',(40.9507912798502,264.245543054191,26.835609378995)) ;
#99899=CARTESIAN_POINT('Ctrl Pts',(41.0160992647417,264.248414211561,26.8085835498115)) ;
#99900=CARTESIAN_POINT('Ctrl Pts',(41.0800412589882,264.251285368931,26.7779876613521)) ;
#99901=CARTESIAN_POINT('Ctrl Pts',(41.1422055473778,264.254156526302,26.7439871588465)) ;
#99902=CARTESIAN_POINT('Ctrl Pts',(41.2027680722295,264.256953703654,26.7108627343366)) ;
#99903=CARTESIAN_POINT('Ctrl Pts',(41.2616429444815,264.259750881006,26.6745072863572)) ;
#99904=CARTESIAN_POINT('Ctrl Pts',(41.3184704556731,264.262548058358,26.6351220940192)) ;
#99905=CARTESIAN_POINT('Ctrl Pts',(41.3752659045721,264.265343657532,26.5957591229528)) ;
#99906=CARTESIAN_POINT('Ctrl Pts',(41.4300158848789,264.268139256706,26.553370076931)) ;
#99907=CARTESIAN_POINT('Ctrl Pts',(41.4823885679606,264.270934855881,26.508200234729)) ;
#99908=CARTESIAN_POINT('Ctrl Pts',(41.5347492659552,264.273729815303,26.4630407292992)) ;
#99909=CARTESIAN_POINT('Ctrl Pts',(41.5847333784703,264.276524774726,26.4151020100271)) ;
#99910=CARTESIAN_POINT('Ctrl Pts',(41.6320425302669,264.279319734149,26.3646693084629)) ;
#99911=CARTESIAN_POINT('Ctrl Pts',(41.6815966902733,264.28224732556,26.3118433737766)) ;
#99912=CARTESIAN_POINT('Ctrl Pts',(41.7282152649853,264.28517491697,26.2562812576092)) ;
#99913=CARTESIAN_POINT('Ctrl Pts',(41.771600737291,264.288102508381,26.1983519372505)) ;
#99914=CARTESIAN_POINT('Ctrl Pts',(41.8130687402515,264.290900711624,26.1429828678253)) ;
#99915=CARTESIAN_POINT('Ctrl Pts',(41.8515831623519,264.293698914866,26.0854518824881)) ;
#99916=CARTESIAN_POINT('Ctrl Pts',(41.8869285156555,264.296497118109,26.0261110844943)) ;
#99917=CARTESIAN_POINT('Ctrl Pts',(41.9222966468408,264.299297124619,25.9667320450475)) ;
#99918=CARTESIAN_POINT('Ctrl Pts',(41.9544914180318,264.30209713113,25.9055413028085)) ;
#99919=CARTESIAN_POINT('Ctrl Pts',(41.9833438858803,264.30489713764,25.8429144250216)) ;
#99920=CARTESIAN_POINT('Ctrl Pts',(42.0122406631827,264.307701444191,25.7801913695777)) ;
#99921=CARTESIAN_POINT('Ctrl Pts',(42.0377847202778,264.310505750741,25.716028231542)) ;
#99922=CARTESIAN_POINT('Ctrl Pts',(42.0598560586647,264.313310057291,25.6508183110292)) ;
#99923=CARTESIAN_POINT('Ctrl Pts',(42.0628488846162,264.31369031522,25.6419759862465)) ;
#99924=CARTESIAN_POINT('Ctrl Pts',(42.0657779348491,264.314070573149,25.6331144322471)) ;
#99925=CARTESIAN_POINT('Ctrl Pts',(42.0686429823233,264.314450831077,25.6242346447783)) ;
#99926=CARTESIAN_POINT('Ctrl Pts',(42.0934907007119,264.317748696824,25.5472228464186)) ;
#99927=CARTESIAN_POINT('Ctrl Pts',(42.1135932196859,264.321046562571,25.4686126575969)) ;
#99928=CARTESIAN_POINT('Ctrl Pts',(42.1287775563013,264.324344428318,25.3889470405068)) ;
#99929=CARTESIAN_POINT('Ctrl Pts',(42.1438184949957,264.327611149663,25.3100337700062)) ;
#99930=CARTESIAN_POINT('Ctrl Pts',(42.1540336338479,264.330877871007,25.2300850204659)) ;
#99931=CARTESIAN_POINT('Ctrl Pts',(42.1593019886856,264.334144592351,25.1496479210032)) ;
#99932=CARTESIAN_POINT('Ctrl Pts',(42.1620665528768,264.33585880127,25.1074386295516)) ;
#99933=CARTESIAN_POINT('Ctrl Pts',(42.1634697555966,264.337573010189,25.0650951796944)) ;
#99934=CARTESIAN_POINT('Ctrl Pts',(42.1634995162458,264.339287219108,25.0226986405015)) ;
#99935=CARTESIAN_POINT('',(42.1634993456137,264.839287219109,25.0197172919184)) ;
#99936=CARTESIAN_POINT('Ctrl Pts',(42.1634995162462,264.33928721913,25.0226986399458)) ;
#99937=CARTESIAN_POINT('Ctrl Pts',(42.1635479241927,264.342075510692,24.9537374350528)) ;
#99938=CARTESIAN_POINT('Ctrl Pts',(42.1599589781167,264.344863802254,24.8847297879806)) ;
#99939=CARTESIAN_POINT('Ctrl Pts',(42.1527445781668,264.347652093816,24.8160866659132)) ;
#99940=CARTESIAN_POINT('Ctrl Pts',(42.1455318298709,264.350439747031,24.7474592589009)) ;
#99941=CARTESIAN_POINT('Ctrl Pts',(42.1346953272965,264.353227400245,24.6791966981854)) ;
#99942=CARTESIAN_POINT('Ctrl Pts',(42.1202988718974,264.35601505346,24.6117052894058)) ;
#99943=CARTESIAN_POINT('Ctrl Pts',(42.1059008215664,264.358803015509,24.5442064034937)) ;
#99944=CARTESIAN_POINT('Ctrl Pts',(42.0879421404037,264.361590977558,24.4774793175867)) ;
#99945=CARTESIAN_POINT('Ctrl Pts',(42.0665374511466,264.364378939607,24.41191883924)) ;
#99946=CARTESIAN_POINT('Ctrl Pts',(42.0451098024302,264.367169892126,24.3462880383052)) ;
#99947=CARTESIAN_POINT('Ctrl Pts',(42.0202289238655,264.369960844646,24.2818268077257)) ;
#99948=CARTESIAN_POINT('Ctrl Pts',(41.9920585786101,264.372751797166,24.2189125290226)) ;
#99949=CARTESIAN_POINT('Ctrl Pts',(41.9638702000318,264.375544536322,24.1559579755733)) ;
#99950=CARTESIAN_POINT('Ctrl Pts',(41.9323883879454,264.378337275477,24.0945527802248)) ;
#99951=CARTESIAN_POINT('Ctrl Pts',(41.8978228576819,264.381130014633,24.0350496941267)) ;
#99952=CARTESIAN_POINT('Ctrl Pts',(41.8632009898797,264.383927305608,23.9754496253585)) ;
#99953=CARTESIAN_POINT('Ctrl Pts',(41.825485645075,264.386724596583,23.9177582595413)) ;
#99954=CARTESIAN_POINT('Ctrl Pts',(41.7849292291823,264.389521887558,23.8622985195703)) ;
#99955=CARTESIAN_POINT('Ctrl Pts',(41.7740574096359,264.390271747772,23.847431616966)) ;
#99956=CARTESIAN_POINT('Ctrl Pts',(41.7629816482407,264.391021607986,23.8327248854236)) ;
#99957=CARTESIAN_POINT('Ctrl Pts',(41.7517072689471,264.3917714682,23.8181841079251)) ;
#99958=CARTESIAN_POINT('Ctrl Pts',(41.7095436440027,264.394575775559,23.7638048935239)) ;
#99959=CARTESIAN_POINT('Ctrl Pts',(41.6644411284693,264.397380082918,23.7115455412584)) ;
#99960=CARTESIAN_POINT('Ctrl Pts',(41.6166405449795,264.400184390277,23.6617388578368)) ;
#99961=CARTESIAN_POINT('Ctrl Pts',(41.5677005192088,264.40305554507,23.6107449119003)) ;
#99962=CARTESIAN_POINT('Ctrl Pts',(41.5159323856718,264.405926699864,23.5623225303253)) ;
#99963=CARTESIAN_POINT('Ctrl Pts',(41.4616400760896,264.408797854657,23.5167949803953)) ;
#99964=CARTESIAN_POINT('Ctrl Pts',(41.4087462681314,264.411595052114,23.4724401629021)) ;
#99965=CARTESIAN_POINT('Ctrl Pts',(41.3534571585366,264.41439224957,23.4308331693213)) ;
#99966=CARTESIAN_POINT('Ctrl Pts',(41.2960911358452,264.417189447027,23.3922357932917)) ;
#99967=CARTESIAN_POINT('Ctrl Pts',(41.2387574840503,264.419985066061,23.3536601972567)) ;
#99968=CARTESIAN_POINT('Ctrl Pts',(41.1793496485779,264.422780685096,23.3180911201278)) ;
#99969=CARTESIAN_POINT('Ctrl Pts',(41.118216854203,264.42557630413,23.2857483748249)) ;
#99970=CARTESIAN_POINT('Ctrl Pts',(41.0570980555312,264.428371283137,23.2534130340496)) ;
#99971=CARTESIAN_POINT('Ctrl Pts',(40.9942555130983,264.431166262145,23.2243027856572)) ;
#99972=CARTESIAN_POINT('Ctrl Pts',(40.9300634902496,264.433961241152,23.1985917432999)) ;
#99973=CARTESIAN_POINT('Ctrl Pts',(40.8628262161465,264.436888813166,23.1716609764268)) ;
#99974=CARTESIAN_POINT('Ctrl Pts',(40.7941087586514,264.43981638518,23.1484602139986)) ;
#99975=CARTESIAN_POINT('Ctrl Pts',(40.7243630542337,264.442743957194,23.1291322880655)) ;
#99976=CARTESIAN_POINT('Ctrl Pts',(40.6576989524889,264.44554217911,23.1106583357027)) ;
#99977=CARTESIAN_POINT('Ctrl Pts',(40.5900960628693,264.448340401025,23.09572225469)) ;
#99978=CARTESIAN_POINT('Ctrl Pts',(40.5219607701516,264.451138622941,23.0843966195882)) ;
#99979=CARTESIAN_POINT('Ctrl Pts',(40.4537815768329,264.453938647793,23.073063687208)) ;
#99980=CARTESIAN_POINT('Ctrl Pts',(40.3850697816922,264.456738672645,23.0653458847321)) ;
#99981=CARTESIAN_POINT('Ctrl Pts',(40.3162366861751,264.459538697498,23.0612638946819)) ;
#99982=CARTESIAN_POINT('Ctrl Pts',(40.2472978972078,264.462343021797,23.0571756367223)) ;
#99983=CARTESIAN_POINT('Ctrl Pts',(40.1782379225077,264.465147346097,23.0567343287291)) ;
#99984=CARTESIAN_POINT('Ctrl Pts',(40.1094667685584,264.467951670397,23.0599086111575)) ;
#99985=CARTESIAN_POINT('Ctrl Pts',(40.1001443772151,264.468331815372,23.0603389064387)) ;
#99986=CARTESIAN_POINT('Ctrl Pts',(40.0908272818648,264.468711960347,23.0608355628873)) ;
#99987=CARTESIAN_POINT('Ctrl Pts',(40.0815164916957,264.469092105321,23.0613984297426)) ;
#99988=CARTESIAN_POINT('Ctrl Pts',(40.0128312227535,264.471896417238,23.0655506725314)) ;
#99989=CARTESIAN_POINT('Ctrl Pts',(39.9442392025349,264.474700729154,23.0733254004651)) ;
#99990=CARTESIAN_POINT('Ctrl Pts',(39.8761510800327,264.477505041071,23.0847114189091)) ;
#99991=CARTESIAN_POINT('Ctrl Pts',(39.8064400399138,264.480376195295,23.0963688293263)) ;
#99992=CARTESIAN_POINT('Ctrl Pts',(39.7372577464111,264.483247349518,23.111811956507)) ;
#99993=CARTESIAN_POINT('Ctrl Pts',(39.669042557486,264.486118503742,23.130972109969)) ;
#99994=CARTESIAN_POINT('Ctrl Pts',(39.6025843513625,264.488915707154,23.1496387654193)) ;
#99995=CARTESIAN_POINT('Ctrl Pts',(39.5370445306828,264.491712910567,23.1718331329916)) ;
#99996=CARTESIAN_POINT('Ctrl Pts',(39.4728188425292,264.494510113979,23.1974399159494)) ;
#99997=CARTESIAN_POINT('Ctrl Pts',(39.4086293846151,264.497305739465,23.2230322539102)) ;
#99998=CARTESIAN_POINT('Ctrl Pts',(39.3457530400132,264.500101364952,23.2520330069956)) ;
#99999=CARTESIAN_POINT('Ctrl Pts',(39.2845682769097,264.502896990439,23.2842777389123)) ;
#100000=CARTESIAN_POINT('Ctrl Pts',(39.2233975108401,264.505691976379,23.3165150943094)) ;
#100001=CARTESIAN_POINT('Ctrl Pts',(39.163917988563,264.50848696232,23.3519947271888)) ;
#100002=CARTESIAN_POINT('Ctrl Pts',(39.1064845590575,264.511281948261,23.3905057524977)) ;
#100003=CARTESIAN_POINT('Ctrl Pts',(39.046326773118,264.514209514443,23.4308435494357)) ;
#100004=CARTESIAN_POINT('Ctrl Pts',(38.9884145298127,264.517137080625,23.4745071981758)) ;
#100005=CARTESIAN_POINT('Ctrl Pts',(38.933120643068,264.520064646807,23.5212040330758)) ;
#100006=CARTESIAN_POINT('Ctrl Pts',(38.8802695713198,264.522862876764,23.5658378600141)) ;
#100007=CARTESIAN_POINT('Ctrl Pts',(38.8298107114831,264.52566110672,23.6132421235063)) ;
#100008=CARTESIAN_POINT('Ctrl Pts',(38.7820331743618,264.528459336677,23.6631221505887)) ;
#100009=CARTESIAN_POINT('Ctrl Pts',(38.734224847177,264.531259369944,23.7130343226767)) ;
#100010=CARTESIAN_POINT('Ctrl Pts',(38.689101599458,264.53405940321,23.7654250646338)) ;
#100011=CARTESIAN_POINT('Ctrl Pts',(38.6469124613425,264.536859436476,23.819966379373)) ;
#100012=CARTESIAN_POINT('Ctrl Pts',(38.6046585349088,264.539663769651,23.8745914512169)) ;
#100013=CARTESIAN_POINT('Ctrl Pts',(38.5653479812375,264.542468102826,23.9313732828279)) ;
#100014=CARTESIAN_POINT('Ctrl Pts',(38.5291861229908,264.545272436001,23.989955597995)) ;
#100015=CARTESIAN_POINT('Ctrl Pts',(38.5242847082473,264.545652538149,23.9978959040852)) ;
#100016=CARTESIAN_POINT('Ctrl Pts',(38.5194410689531,264.546032640296,24.0058692530938)) ;
#100017=CARTESIAN_POINT('Ctrl Pts',(38.5146556495777,264.546412742443,24.0138747269133)) ;
#100018=CARTESIAN_POINT('Ctrl Pts',(38.4793526268504,264.549216834142,24.0729327533947)) ;
#100019=CARTESIAN_POINT('Ctrl Pts',(38.4470931245889,264.552020925841,24.1339564703419)) ;
#100020=CARTESIAN_POINT('Ctrl Pts',(38.4180994832558,264.554825017539,24.196600513298)) ;
#100021=CARTESIAN_POINT('Ctrl Pts',(38.3884121467348,264.55769619929,24.2607433632047)) ;
#100022=CARTESIAN_POINT('Ctrl Pts',(38.3621493053107,264.560567381041,24.3265846793667)) ;
#100023=CARTESIAN_POINT('Ctrl Pts',(38.3395014964272,264.563438562793,24.3937236831134)) ;
#100024=CARTESIAN_POINT('Ctrl Pts',(38.3174389729793,264.566235544833,24.459127619187)) ;
#100025=CARTESIAN_POINT('Ctrl Pts',(38.2988070560149,264.569032526874,24.5257624869819)) ;
#100026=CARTESIAN_POINT('Ctrl Pts',(38.283733713274,264.571829508914,24.5932365102311)) ;
#100027=CARTESIAN_POINT('Ctrl Pts',(38.2686688730836,264.574624913237,24.6606724728257)) ;
#100028=CARTESIAN_POINT('Ctrl Pts',(38.2571587297346,264.57742031756,24.7289461766327)) ;
#100029=CARTESIAN_POINT('Ctrl Pts',(38.2492809271652,264.580215721883,24.7976524002183)) ;
#100030=CARTESIAN_POINT('Ctrl Pts',(38.2414049252721,264.583010487243,24.8663429192128)) ;
#100031=CARTESIAN_POINT('Ctrl Pts',(38.2371596703656,264.585805252604,24.9354652774667)) ;
#100032=CARTESIAN_POINT('Ctrl Pts',(38.2365711286217,264.588600017965,25.0046075628753)) ;
#100033=CARTESIAN_POINT('Ctrl Pts',(38.2359545756725,264.591527798098,25.0770406237873)) ;
#100034=CARTESIAN_POINT('Ctrl Pts',(38.2393515526775,264.594455578231,25.1494949762986)) ;
#100035=CARTESIAN_POINT('Ctrl Pts',(38.2467306029344,264.597383358365,25.2214975462755)) ;
#100036=CARTESIAN_POINT('Ctrl Pts',(38.2537825947889,264.600181371786,25.2903087779779)) ;
#100037=CARTESIAN_POINT('Ctrl Pts',(38.2644709950671,264.602979385207,25.3587069333941)) ;
#100038=CARTESIAN_POINT('Ctrl Pts',(38.2787154960898,264.605777398627,25.4262871385375)) ;
#100039=CARTESIAN_POINT('Ctrl Pts',(38.2929691857925,264.608577216959,25.4939109375475)) ;
#100040=CARTESIAN_POINT('Ctrl Pts',(38.3107834159673,264.61137703529,25.5607152655708)) ;
#100041=CARTESIAN_POINT('Ctrl Pts',(38.3320277571629,264.614176853622,25.6263095583315)) ;
#100042=CARTESIAN_POINT('Ctrl Pts',(38.35330475354,264.61698097562,25.6920046776376)) ;
#100043=CARTESIAN_POINT('Ctrl Pts',(38.3780222024389,264.619785097619,25.7564855981368)) ;
#100044=CARTESIAN_POINT('Ctrl Pts',(38.4060016741804,264.622589219618,25.8193819056941)) ;
#100045=CARTESIAN_POINT('Ctrl Pts',(38.409807142338,264.622970606267,25.8279363879891)) ;
#100046=CARTESIAN_POINT('Ctrl Pts',(38.4136728845381,264.623351992916,25.8364615962601)) ;
#100047=CARTESIAN_POINT('Ctrl Pts',(38.4175983879456,264.623733379566,25.8449566366805)) ;
#100048=CARTESIAN_POINT('Ctrl Pts',(38.4464655112008,264.62653799703,25.9074269375343)) ;
#100049=CARTESIAN_POINT('Ctrl Pts',(38.4786733892577,264.629342614494,25.9684916631513)) ;
#100050=CARTESIAN_POINT('Ctrl Pts',(38.5140620943109,264.632147231958,26.0277723434883)) ;
#100051=CARTESIAN_POINT('Ctrl Pts',(38.550289879267,264.635018347988,26.0884585917157)) ;
#100052=CARTESIAN_POINT('Ctrl Pts',(38.589851123995,264.637889464019,26.1472746073566)) ;
#100053=CARTESIAN_POINT('Ctrl Pts',(38.6325223457163,264.640760580049,26.2038371735969)) ;
#100054=CARTESIAN_POINT('Ctrl Pts',(38.6740995212223,264.643558083619,26.2589495338428)) ;
#100055=CARTESIAN_POINT('Ctrl Pts',(38.7186287952341,264.646355587189,26.3119221999099)) ;
#100056=CARTESIAN_POINT('Ctrl Pts',(38.7658587081481,264.649153090759,26.3624284693292)) ;
#100057=CARTESIAN_POINT('Ctrl Pts',(38.8130619331503,264.651949013561,26.4129061994865)) ;
#100058=CARTESIAN_POINT('Ctrl Pts',(38.8629624364252,264.654744936363,26.4609199434834)) ;
#100059=CARTESIAN_POINT('Ctrl Pts',(38.9152692766348,264.657540859165,26.5061769758449)) ;
#100060=CARTESIAN_POINT('Ctrl Pts',(38.9675640897254,264.660336139089,26.5514236020776)) ;
#100061=CARTESIAN_POINT('Ctrl Pts',(39.0222637722745,264.663131419014,26.593914457129)) ;
#100062=CARTESIAN_POINT('Ctrl Pts',(39.0790427136724,264.665926698938,26.633395717799)) ;
#100063=CARTESIAN_POINT('Ctrl Pts',(39.1385028264927,264.668853975417,26.6747413321399)) ;
#100064=CARTESIAN_POINT('Ctrl Pts',(39.20024298406,264.671781251896,26.7127857088493)) ;
#100065=CARTESIAN_POINT('Ctrl Pts',(39.2638551061375,264.674708528376,26.7472881844231)) ;
#100066=CARTESIAN_POINT('Ctrl Pts',(39.3246690750271,264.677507040592,26.7802729742342)) ;
#100067=CARTESIAN_POINT('Ctrl Pts',(39.3871932902662,264.680305552808,26.810020760495)) ;
#100068=CARTESIAN_POINT('Ctrl Pts',(39.4510480207014,264.683104065025,26.8363694290404)) ;
#100069=CARTESIAN_POINT('Ctrl Pts',(39.5149437996222,264.685904376241,26.8627350356096)) ;
#100070=CARTESIAN_POINT('Ctrl Pts',(39.5801713366973,264.688704687458,26.8856970140323)) ;
#100071=CARTESIAN_POINT('Ctrl Pts',(39.6463344402367,264.691504998675,26.9051427072479)) ;
#100072=CARTESIAN_POINT('Ctrl Pts',(39.7125989490608,264.694309601806,26.9246182040238)) ;
#100073=CARTESIAN_POINT('Ctrl Pts',(39.7798014112819,264.697114204936,26.9405665548798)) ;
#100074=CARTESIAN_POINT('Ctrl Pts',(39.8475351930882,264.699918808067,26.9529261029962)) ;
#100075=CARTESIAN_POINT('Ctrl Pts',(39.8566739754725,264.700297210941,26.9545936788733)) ;
#100076=CARTESIAN_POINT('Ctrl Pts',(39.8658224235725,264.700675613815,26.9561960016907)) ;
#100077=CARTESIAN_POINT('Ctrl Pts',(39.8749795341706,264.701054016688,26.9577329924524)) ;
#100078=CARTESIAN_POINT('Ctrl Pts',(39.9428436807735,264.703858393443,26.9691237652583)) ;
#100079=CARTESIAN_POINT('Ctrl Pts',(40.0114309987808,264.706662770198,26.9769634518271)) ;
#100080=CARTESIAN_POINT('Ctrl Pts',(40.0803387932757,264.709467146952,26.9811707066244)) ;
#100081=CARTESIAN_POINT('Ctrl Pts',(40.150887212427,264.712338293071,26.9854781318887)) ;
#100082=CARTESIAN_POINT('Ctrl Pts',(40.2217710722778,264.71520943919,26.9859777612121)) ;
#100083=CARTESIAN_POINT('Ctrl Pts',(40.2925477963527,264.71808058531,26.9826380524967)) ;
#100084=CARTESIAN_POINT('Ctrl Pts',(40.3615035625385,264.720877862,26.9793842684834)) ;
#100085=CARTESIAN_POINT('Ctrl Pts',(40.4303571204035,264.72367513869,26.9724863577426)) ;
#100086=CARTESIAN_POINT('Ctrl Pts',(40.4986969110173,264.726472415381,26.9619677626826)) ;
#100087=CARTESIAN_POINT('Ctrl Pts',(40.5669982215106,264.729268117007,26.9514550903333)) ;
#100088=CARTESIAN_POINT('Ctrl Pts',(40.634785858032,264.732063818633,26.9373258534575)) ;
#100089=CARTESIAN_POINT('Ctrl Pts',(40.7016540599149,264.73485952026,26.9196552597878)) ;
#100090=CARTESIAN_POINT('Ctrl Pts',(40.7685070292218,264.737654585025,26.9019886914791)) ;
#100091=CARTESIAN_POINT('Ctrl Pts',(40.8344405089517,264.740449649791,26.8807824933933)) ;
#100092=CARTESIAN_POINT('Ctrl Pts',(40.8990613189203,264.743244714556,26.8561624409591)) ;
#100093=CARTESIAN_POINT('Ctrl Pts',(40.9667438629519,264.746172209494,26.8303758904076)) ;
#100094=CARTESIAN_POINT('Ctrl Pts',(41.0329856991877,264.749099704432,26.8008441120265)) ;
#100095=CARTESIAN_POINT('Ctrl Pts',(41.0973578329321,264.75202719937,26.7677685018727)) ;
#100096=CARTESIAN_POINT('Ctrl Pts',(41.1588894396531,264.754825513744,26.7361524078014)) ;
#100097=CARTESIAN_POINT('Ctrl Pts',(41.218712467216,264.757623828119,26.7012989621997)) ;
#100098=CARTESIAN_POINT('Ctrl Pts',(41.2764789663989,264.760422142494,26.663430353547)) ;
#100099=CARTESIAN_POINT('Ctrl Pts',(41.3342827293884,264.763222261995,26.6255373167477)) ;
#100100=CARTESIAN_POINT('Ctrl Pts',(41.3900269312364,264.766022381497,26.5846255341491)) ;
#100101=CARTESIAN_POINT('Ctrl Pts',(41.4433951909114,264.768822500998,26.5409586719846)) ;
#100102=CARTESIAN_POINT('Ctrl Pts',(41.4968454397676,264.771626922298,26.4972247248094)) ;
#100103=CARTESIAN_POINT('Ctrl Pts',(41.5479121071341,264.774431343598,26.4507275837462)) ;
#100104=CARTESIAN_POINT('Ctrl Pts',(41.5963150473167,264.777235764898,26.4017682921028)) ;
#100105=CARTESIAN_POINT('Ctrl Pts',(41.6028672692048,264.777615394536,26.3951407578843)) ;
#100106=CARTESIAN_POINT('Ctrl Pts',(41.6093707401449,264.777995024173,26.3884681550574)) ;
#100107=CARTESIAN_POINT('Ctrl Pts',(41.6158248231222,264.77837465381,26.3817512753716)) ;
#100108=CARTESIAN_POINT('Ctrl Pts',(41.6628292052529,264.781139455038,26.3328329734866)) ;
#100109=CARTESIAN_POINT('Ctrl Pts',(41.7073932893235,264.783904256266,26.2813735376347)) ;
#100110=CARTESIAN_POINT('Ctrl Pts',(41.7492265774585,264.786669057493,26.2276491800284)) ;
#100111=CARTESIAN_POINT('Ctrl Pts',(41.7910060149023,264.789430299679,26.1739939801174)) ;
#100112=CARTESIAN_POINT('Ctrl Pts',(41.8300613170704,264.792191541864,26.1180800296299)) ;
#100113=CARTESIAN_POINT('Ctrl Pts',(41.8661394144824,264.794952784049,26.060219617555)) ;
#100114=CARTESIAN_POINT('Ctrl Pts',(41.9021840563867,264.797711465712,26.0024128599022)) ;
#100115=CARTESIAN_POINT('Ctrl Pts',(41.9352567027741,264.800470147375,25.9426636440052)) ;
#100116=CARTESIAN_POINT('Ctrl Pts',(41.9651463200989,264.803228829038,25.8813149474039)) ;
#100117=CARTESIAN_POINT('Ctrl Pts',(41.9950189755122,264.805985945191,25.8200010652719)) ;
#100118=CARTESIAN_POINT('Ctrl Pts',(42.0217119664681,264.808743061343,25.757089954604)) ;
#100119=CARTESIAN_POINT('Ctrl Pts',(42.0450601063211,264.811500177496,25.6929492992057)) ;
#100120=CARTESIAN_POINT('Ctrl Pts',(42.0684116860251,264.81425769985,25.6287991940485)) ;
#100121=CARTESIAN_POINT('Ctrl Pts',(42.0884172473216,264.817015222205,25.5634196508713)) ;
#100122=CARTESIAN_POINT('Ctrl Pts',(42.1049602730527,264.81977274456,25.4971970167546)) ;
#100123=CARTESIAN_POINT('Ctrl Pts',(42.1215047963007,264.822530516533,25.4309683879956)) ;
#100124=CARTESIAN_POINT('Ctrl Pts',(42.1345860514729,264.825288288506,25.3638970075198)) ;
#100125=CARTESIAN_POINT('Ctrl Pts',(42.1441383952741,264.828046060479,25.2963806097214)) ;
#100126=CARTESIAN_POINT('Ctrl Pts',(42.1536997060346,264.830806421222,25.2288008330492)) ;
#100127=CARTESIAN_POINT('Ctrl Pts',(42.1597254422429,264.833566781966,25.1607757055302)) ;
#100128=CARTESIAN_POINT('Ctrl Pts',(42.1622018410338,264.83632714271,25.0927079128119)) ;
#100129=CARTESIAN_POINT('Ctrl Pts',(42.1630870308451,264.837313834843,25.0683770510719)) ;
#100130=CARTESIAN_POINT('Ctrl Pts',(42.1635192039033,264.838300526976,25.0440407370176)) ;
#100131=CARTESIAN_POINT('Ctrl Pts',(42.1634993456137,264.839287219109,25.0197172919184)) ;
#100132=CARTESIAN_POINT('',(39.3481011574342,264.999957040867,23.2522526195775)) ;
#100133=CARTESIAN_POINT('Ctrl Pts',(42.1634993456133,264.83928721913,25.0197172914112)) ;
#100134=CARTESIAN_POINT('Ctrl Pts',(42.1634231064844,264.843075285805,24.9263357505314)) ;
#100135=CARTESIAN_POINT('Ctrl Pts',(42.1566814593656,264.846863352479,24.833221909536)) ;
#100136=CARTESIAN_POINT('Ctrl Pts',(42.1434103250307,264.850651419153,24.7411622478992)) ;
#100137=CARTESIAN_POINT('Ctrl Pts',(42.1375200820027,264.852332709746,24.7003026072363)) ;
#100138=CARTESIAN_POINT('Ctrl Pts',(42.1303441968703,264.854014000339,24.6596502838563)) ;
#100139=CARTESIAN_POINT('Ctrl Pts',(42.1218974742994,264.855695290932,24.6192726495211)) ;
#100140=CARTESIAN_POINT('Ctrl Pts',(42.1077899698027,264.858503340374,24.5518349358796)) ;
#100141=CARTESIAN_POINT('Ctrl Pts',(42.0901033726998,264.861311389816,24.4850193578663)) ;
#100142=CARTESIAN_POINT('Ctrl Pts',(42.0689090738205,264.864119439258,24.4192313768849)) ;
#100143=CARTESIAN_POINT('Ctrl Pts',(42.0472420055495,264.866990126291,24.3519759001431)) ;
#100144=CARTESIAN_POINT('Ctrl Pts',(42.0219088766885,264.869860813324,24.2857949364322)) ;
#100145=CARTESIAN_POINT('Ctrl Pts',(41.9930413906057,264.872731500357,24.2211111074377)) ;
#100146=CARTESIAN_POINT('Ctrl Pts',(41.9648754428109,264.87553242389,24.1579992262922)) ;
#100147=CARTESIAN_POINT('Ctrl Pts',(41.9333451893783,264.878333347424,24.0963130074087)) ;
#100148=CARTESIAN_POINT('Ctrl Pts',(41.8986227463113,264.881134270957,24.0364279556745)) ;
#100149=CARTESIAN_POINT('Ctrl Pts',(41.8639200754108,264.883933599547,23.9765770045713)) ;
#100150=CARTESIAN_POINT('Ctrl Pts',(41.8260290658077,264.886732928136,23.9185256046506)) ;
#100151=CARTESIAN_POINT('Ctrl Pts',(41.7851679310898,264.889532256726,23.862625008174)) ;
#100152=CARTESIAN_POINT('Ctrl Pts',(41.7443164700062,264.892330922592,23.8067376458361)) ;
#100153=CARTESIAN_POINT('Ctrl Pts',(41.7004965673578,264.895129588457,23.7530004675247)) ;
#100154=CARTESIAN_POINT('Ctrl Pts',(41.6539689599815,264.897928254322,23.7017346080311)) ;
#100155=CARTESIAN_POINT('Ctrl Pts',(41.605358134152,264.900852227133,23.6481733804638)) ;
#100156=CARTESIAN_POINT('Ctrl Pts',(41.5537917794676,264.903776199944,23.5973104348385)) ;
#100157=CARTESIAN_POINT('Ctrl Pts',(41.4996115905637,264.906700172755,23.5494704994273)) ;
#100158=CARTESIAN_POINT('Ctrl Pts',(41.4476950435001,264.90950198233,23.5036293108204)) ;
#100159=CARTESIAN_POINT('Ctrl Pts',(41.3933791649083,264.912303791906,23.4605638234563)) ;
#100160=CARTESIAN_POINT('Ctrl Pts',(41.3369979930227,264.915105601481,23.4205181028495)) ;
#100161=CARTESIAN_POINT('Ctrl Pts',(41.2805812983321,264.917909176329,23.3804471515447)) ;
#100162=CARTESIAN_POINT('Ctrl Pts',(41.2220971304581,264.920712751176,23.3434000140179)) ;
#100163=CARTESIAN_POINT('Ctrl Pts',(41.1619067425903,264.923516326024,23.3095763006141)) ;
#100164=CARTESIAN_POINT('Ctrl Pts',(41.101625711966,264.926324122871,23.2757016509276)) ;
#100165=CARTESIAN_POINT('Ctrl Pts',(41.039633771008,264.929131919718,23.2450603222638)) ;
#100166=CARTESIAN_POINT('Ctrl Pts',(40.9763138793755,264.931939716564,23.2178046073685)) ;
#100167=CARTESIAN_POINT('Ctrl Pts',(40.9682238359863,264.932298453728,23.214322290668)) ;
#100168=CARTESIAN_POINT('Ctrl Pts',(40.9601121367656,264.932657190891,23.2108951736593)) ;
#100169=CARTESIAN_POINT('Ctrl Pts',(40.9519795979876,264.933015928055,23.2075235152984)) ;
#100170=CARTESIAN_POINT('Ctrl Pts',(40.8887483928988,264.935805141089,23.18130857466)) ;
#100171=CARTESIAN_POINT('Ctrl Pts',(40.8240121001998,264.938594354122,23.1583492976769)) ;
#100172=CARTESIAN_POINT('Ctrl Pts',(40.7581442156735,264.941383567156,23.1388200687893)) ;
#100173=CARTESIAN_POINT('Ctrl Pts',(40.6930035405595,264.944141986094,23.1195064508806)) ;
#100174=CARTESIAN_POINT('Ctrl Pts',(40.6267566189771,264.946900405032,23.1035476997139)) ;
#100175=CARTESIAN_POINT('Ctrl Pts',(40.5597860729364,264.949658823969,23.0910648600235)) ;
#100176=CARTESIAN_POINT('Ctrl Pts',(40.4928740653508,264.952414831794,23.0785929314903)) ;
#100177=CARTESIAN_POINT('Ctrl Pts',(40.4252401800672,264.955170839618,23.0695909839479)) ;
#100178=CARTESIAN_POINT('Ctrl Pts',(40.3572802186558,264.957926847442,23.0641297082817)) ;
#100179=CARTESIAN_POINT('Ctrl Pts',(40.2893551072405,264.96068144198,23.0586712331679)) ;
#100180=CARTESIAN_POINT('Ctrl Pts',(40.2211047526861,264.963436036518,23.0567498687277)) ;
#100181=CARTESIAN_POINT('Ctrl Pts',(40.1529311591549,264.966190631057,23.0583845895876)) ;
#100182=CARTESIAN_POINT('Ctrl Pts',(40.0832906166155,264.969004498541,23.0600544861222)) ;
#100183=CARTESIAN_POINT('Ctrl Pts',(40.0137307198484,264.971818366025,23.0654353438013)) ;
#100184=CARTESIAN_POINT('Ctrl Pts',(39.9446791624989,264.974632233509,23.0744912498953)) ;
#100185=CARTESIAN_POINT('Ctrl Pts',(39.8770450615677,264.977388339305,23.0833612608016)) ;
#100186=CARTESIAN_POINT('Ctrl Pts',(39.8098991283124,264.980144445101,23.0957567194047)) ;
#100187=CARTESIAN_POINT('Ctrl Pts',(39.743634804907,264.982900550897,23.1115918134518)) ;
#100188=CARTESIAN_POINT('Ctrl Pts',(39.6752873579909,264.985743299225,23.1279247086535)) ;
#100189=CARTESIAN_POINT('Ctrl Pts',(39.6078784423246,264.988586047554,23.1479169980995)) ;
#100190=CARTESIAN_POINT('Ctrl Pts',(39.5418221791217,264.991428795882,23.1714192094165)) ;
#100191=CARTESIAN_POINT('Ctrl Pts',(39.4757659159188,264.99427154421,23.1949214207335)) ;
#100192=CARTESIAN_POINT('Ctrl Pts',(39.4110628212892,264.997114292539,23.2219332780187)) ;
#100193=CARTESIAN_POINT('Ctrl Pts',(39.3481011574342,264.999957040867,23.2522526195775)) ;
#100194=CARTESIAN_POINT('',(41.0518972680585,265.,23.2522518613707)) ;
#100195=CARTESIAN_POINT('Origin',(40.2,265.,25.0213203435596)) ;
#100196=CARTESIAN_POINT('',(42.1634997790836,264.91071278087,25.0203889259126)) ;
#100197=CARTESIAN_POINT('Ctrl Pts',(41.0518972680585,265.,23.2522518613707)) ;
#100198=CARTESIAN_POINT('Ctrl Pts',(41.6248630396448,264.974226454293,23.5281642867062)) ;
#100199=CARTESIAN_POINT('Ctrl Pts',(42.1146717303696,264.944464047916,24.1908662058816)) ;
#100200=CARTESIAN_POINT('Ctrl Pts',(42.1650160107952,264.914701641539,24.9222347032997)) ;
#100201=CARTESIAN_POINT('Ctrl Pts',(42.1642443780331,264.91071278087,25.0203885727001)) ;
#100202=CARTESIAN_POINT('',(42.1634997239514,264.410712780843,25.0223615172765)) ;
#100203=CARTESIAN_POINT('Ctrl Pts',(42.1634997790836,264.91071278087,25.0203889259126)) ;
#100204=CARTESIAN_POINT('Ctrl Pts',(42.1635318794642,264.907961693408,25.08805898823)) ;
#100205=CARTESIAN_POINT('Ctrl Pts',(42.1600614472557,264.905210605947,25.1558539686729)) ;
#100206=CARTESIAN_POINT('Ctrl Pts',(42.1530760488447,264.902459518485,25.2233752802212)) ;
#100207=CARTESIAN_POINT('Ctrl Pts',(42.1460976350027,264.899711181784,25.2908290784746)) ;
#100208=CARTESIAN_POINT('Ctrl Pts',(42.1356112693631,264.896962845084,25.3580092487036)) ;
#100209=CARTESIAN_POINT('Ctrl Pts',(42.1216565407332,264.894214508383,25.4245180487331)) ;
#100210=CARTESIAN_POINT('Ctrl Pts',(42.1077106617737,264.891467914595,25.4909846708768)) ;
#100211=CARTESIAN_POINT('Ctrl Pts',(42.0903008831812,264.888721320807,25.5567802716991)) ;
#100212=CARTESIAN_POINT('Ctrl Pts',(42.0695182592163,264.885974727019,25.6215150856698)) ;
#100213=CARTESIAN_POINT('Ctrl Pts',(42.0487412166764,264.883228870862,25.6862325143235)) ;
#100214=CARTESIAN_POINT('Ctrl Pts',(42.0245932812702,264.880483014705,25.7498892389648)) ;
#100215=CARTESIAN_POINT('Ctrl Pts',(41.9972154150436,264.877737158547,25.8121104559975)) ;
#100216=CARTESIAN_POINT('Ctrl Pts',(41.9698165503494,264.874989196354,25.8743793958953)) ;
#100217=CARTESIAN_POINT('Ctrl Pts',(41.9391830068083,264.872241234161,25.9352101618639)) ;
#100218=CARTESIAN_POINT('Ctrl Pts',(41.9055035211403,264.869493271968,25.9942489069075)) ;
#100219=CARTESIAN_POINT('Ctrl Pts',(41.8718123184394,264.866744353764,26.0533081914247)) ;
#100220=CARTESIAN_POINT('Ctrl Pts',(41.8350733360558,264.86399543556,26.1105737849847)) ;
#100221=CARTESIAN_POINT('Ctrl Pts',(41.795519279112,264.861246517355,26.1657199590707)) ;
#100222=CARTESIAN_POINT('Ctrl Pts',(41.7558956597364,264.858492764718,26.2209631169371)) ;
#100223=CARTESIAN_POINT('Ctrl Pts',(41.7134473926541,264.855739012081,26.2740790117971)) ;
#100224=CARTESIAN_POINT('Ctrl Pts',(41.6684476868165,264.852985259444,26.3247748464416)) ;
#100225=CARTESIAN_POINT('Ctrl Pts',(41.6269053725341,264.850443081548,26.3715756478337)) ;
#100226=CARTESIAN_POINT('Ctrl Pts',(41.5831892778027,264.847900903652,26.4163141561029)) ;
#100227=CARTESIAN_POINT('Ctrl Pts',(41.537539930606,264.845358725756,26.4587900594265)) ;
#100228=CARTESIAN_POINT('Ctrl Pts',(41.4871947620435,264.842555041091,26.505635340772)) ;
#100229=CARTESIAN_POINT('Ctrl Pts',(41.4342916268096,264.839751356426,26.5499200365583)) ;
#100230=CARTESIAN_POINT('Ctrl Pts',(41.3791209197052,264.836947671762,26.591354135143)) ;
#100231=CARTESIAN_POINT('Ctrl Pts',(41.3226210085465,264.834076439131,26.6337864875967)) ;
#100232=CARTESIAN_POINT('Ctrl Pts',(41.2637431565371,264.831205206501,26.6732286841668)) ;
#100233=CARTESIAN_POINT('Ctrl Pts',(41.2028388445095,264.828333973871,26.7094099448376)) ;
#100234=CARTESIAN_POINT('Ctrl Pts',(41.1435228607675,264.825537620339,26.7446476316)) ;
#100235=CARTESIAN_POINT('Ctrl Pts',(41.0822852734038,264.822741266808,26.7767921278507)) ;
#100236=CARTESIAN_POINT('Ctrl Pts',(41.0194817836898,264.819944913276,26.8056358583161)) ;
#100237=CARTESIAN_POINT('Ctrl Pts',(40.9567155109527,264.817150216847,26.8344624961572)) ;
#100238=CARTESIAN_POINT('Ctrl Pts',(40.8923856197779,264.814355520418,26.8599920465211)) ;
#100239=CARTESIAN_POINT('Ctrl Pts',(40.8268715866425,264.811560823989,26.8820632768688)) ;
#100240=CARTESIAN_POINT('Ctrl Pts',(40.7613743468544,264.808766843931,26.9041288496526)) ;
#100241=CARTESIAN_POINT('Ctrl Pts',(40.6946940301555,264.805972863872,26.9227377074936)) ;
#100242=CARTESIAN_POINT('Ctrl Pts',(40.6272275679252,264.803178883814,26.9377777146495)) ;
#100243=CARTESIAN_POINT('Ctrl Pts',(40.5565152662079,264.800250484215,26.9535413027891)) ;
#100244=CARTESIAN_POINT('Ctrl Pts',(40.4849398237965,264.797322084617,26.9653838072331)) ;
#100245=CARTESIAN_POINT('Ctrl Pts',(40.4129707807618,264.794393685019,26.9732362476246)) ;
#100246=CARTESIAN_POINT('Ctrl Pts',(40.3442299014721,264.791596638472,26.9807364676402)) ;
#100247=CARTESIAN_POINT('Ctrl Pts',(40.2751304898507,264.788799591925,26.984596937117)) ;
#100248=CARTESIAN_POINT('Ctrl Pts',(40.206085015493,264.786002545378,26.9848109146056)) ;
#100249=CARTESIAN_POINT('Ctrl Pts',(40.1369964994812,264.783203755205,26.9850250254837)) ;
#100250=CARTESIAN_POINT('Ctrl Pts',(40.0679624746254,264.780404965032,26.9815881443537)) ;
#100251=CARTESIAN_POINT('Ctrl Pts',(39.9993919948402,264.777606174858,26.9745455426254)) ;
#100252=CARTESIAN_POINT('Ctrl Pts',(39.9307179913896,264.774803159237,26.9674923083926)) ;
#100253=CARTESIAN_POINT('Ctrl Pts',(39.8625094096421,264.772000143615,26.9568225715688)) ;
#100254=CARTESIAN_POINT('Ctrl Pts',(39.7951657177126,264.769197127994,26.9426327736149)) ;
#100255=CARTESIAN_POINT('Ctrl Pts',(39.7858835730344,264.76881078154,26.9406769592871)) ;
#100256=CARTESIAN_POINT('Ctrl Pts',(39.776617835104,264.768424435087,26.9386543488758)) ;
#100257=CARTESIAN_POINT('Ctrl Pts',(39.7673695251547,264.768038088634,26.9365652684283)) ;
#100258=CARTESIAN_POINT('Ctrl Pts',(39.7001575510037,264.76523032073,26.9213829030218)) ;
#100259=CARTESIAN_POINT('Ctrl Pts',(39.6336264701506,264.762422552827,26.902631367906)) ;
#100260=CARTESIAN_POINT('Ctrl Pts',(39.5681805075374,264.759614784923,26.8803890294731)) ;
#100261=CARTESIAN_POINT('Ctrl Pts',(39.501267149348,264.756744062698,26.8576479848143)) ;
#100262=CARTESIAN_POINT('Ctrl Pts',(39.4354886779217,264.753873340472,26.8312577286187)) ;
#100263=CARTESIAN_POINT('Ctrl Pts',(39.3712655380563,264.751002618247,26.8013572649708)) ;
#100264=CARTESIAN_POINT('Ctrl Pts',(39.3086065396949,264.748201811877,26.7721850210311)) ;
#100265=CARTESIAN_POINT('Ctrl Pts',(39.2474284393559,264.745401005507,26.7396718313736)) ;
#100266=CARTESIAN_POINT('Ctrl Pts',(39.1881037596738,264.742600199137,26.7039962626877)) ;
#100267=CARTESIAN_POINT('Ctrl Pts',(39.1288115674895,264.739800926551,26.668340230727)) ;
#100268=CARTESIAN_POINT('Ctrl Pts',(39.0713711972851,264.737001653964,26.629525506797)) ;
#100269=CARTESIAN_POINT('Ctrl Pts',(39.016130114285,264.734202381377,26.5877763256086)) ;
#100270=CARTESIAN_POINT('Ctrl Pts',(38.9609009043902,264.731403710445,26.5460361176771)) ;
#100271=CARTESIAN_POINT('Ctrl Pts',(38.9078704301041,264.728605039513,26.5013629984539)) ;
#100272=CARTESIAN_POINT('Ctrl Pts',(38.8573552983472,264.725806368581,26.4540231931148)) ;
#100273=CARTESIAN_POINT('Ctrl Pts',(38.8045766368541,264.722882292159,26.4045621410648)) ;
#100274=CARTESIAN_POINT('Ctrl Pts',(38.7545444947112,264.719958215736,26.352190151185)) ;
#100275=CARTESIAN_POINT('Ctrl Pts',(38.7075776766873,264.717034139314,26.2972544558389)) ;
#100276=CARTESIAN_POINT('Ctrl Pts',(38.6625721943867,264.71423217241,26.2446128767711)) ;
#100277=CARTESIAN_POINT('Ctrl Pts',(38.6203813700412,264.711430205506,26.1896178964985)) ;
#100278=CARTESIAN_POINT('Ctrl Pts',(38.5812434763964,264.708628238603,26.1326076904194)) ;
#100279=CARTESIAN_POINT('Ctrl Pts',(38.5420801920694,264.705824453925,26.0755604990074)) ;
#100280=CARTESIAN_POINT('Ctrl Pts',(38.505974033711,264.703020669247,26.0164958939749)) ;
#100281=CARTESIAN_POINT('Ctrl Pts',(38.4731183471652,264.700216884569,25.9557784791134)) ;
#100282=CARTESIAN_POINT('Ctrl Pts',(38.440212338251,264.697408805563,25.8949680683523)) ;
#100283=CARTESIAN_POINT('Ctrl Pts',(38.4105669385035,264.694600726558,25.832500236649)) ;
#100284=CARTESIAN_POINT('Ctrl Pts',(38.38432780638,264.691792647552,25.7687604651179)) ;
#100285=CARTESIAN_POINT('Ctrl Pts',(38.3809788727128,264.691434248872,25.7606252773452)) ;
#100286=CARTESIAN_POINT('Ctrl Pts',(38.3776853596183,264.691075850192,25.7524693901348)) ;
#100287=CARTESIAN_POINT('Ctrl Pts',(38.3744475111506,264.690717451512,25.7442936213892)) ;
#100288=CARTESIAN_POINT('Ctrl Pts',(38.3491290417838,264.687914940494,25.6803629116608)) ;
#100289=CARTESIAN_POINT('Ctrl Pts',(38.3271260734493,264.685112429476,25.6149825030002)) ;
#100290=CARTESIAN_POINT('Ctrl Pts',(38.3086026758496,264.682309918458,25.5485284734257)) ;
#100291=CARTESIAN_POINT('Ctrl Pts',(38.2896240881604,264.679438539122,25.4804414164589)) ;
#100292=CARTESIAN_POINT('Ctrl Pts',(38.2742986221662,264.676567159786,25.4112277197905)) ;
#100293=CARTESIAN_POINT('Ctrl Pts',(38.2627503035205,264.673695780449,25.3413138801974)) ;
#100294=CARTESIAN_POINT('Ctrl Pts',(38.2515077943795,264.670900437731,25.2732514197807)) ;
#100295=CARTESIAN_POINT('Ctrl Pts',(38.2438449491744,264.668105095013,25.2045259531586)) ;
#100296=CARTESIAN_POINT('Ctrl Pts',(38.239825227063,264.665309752295,25.1355442882526)) ;
#100297=CARTESIAN_POINT('Ctrl Pts',(38.2358077982496,264.662516004352,25.066601978187)) ;
#100298=CARTESIAN_POINT('Ctrl Pts',(38.2354293964421,264.659722256409,24.9974042463009)) ;
#100299=CARTESIAN_POINT('Ctrl Pts',(38.2387016537863,264.656928508466,24.9283631107076)) ;
#100300=CARTESIAN_POINT('Ctrl Pts',(38.2419731460447,264.654135413729,24.8593381176099)) ;
#100301=CARTESIAN_POINT('Ctrl Pts',(38.2488935788787,264.651342318992,24.7904701354936)) ;
#100302=CARTESIAN_POINT('Ctrl Pts',(38.2594225028232,264.648549224255,24.7221694995843)) ;
#100303=CARTESIAN_POINT('Ctrl Pts',(38.2704651241443,264.645619856766,24.6505365328817)) ;
#100304=CARTESIAN_POINT('Ctrl Pts',(38.2854773069324,264.642690489278,24.5795282721564)) ;
#100305=CARTESIAN_POINT('Ctrl Pts',(38.3043517094858,264.639761121789,24.5096077204295)) ;
#100306=CARTESIAN_POINT('Ctrl Pts',(38.3223689069501,264.636964795265,24.4428626998276)) ;
#100307=CARTESIAN_POINT('Ctrl Pts',(38.3439049015649,264.63416846874,24.3771091994739)) ;
#100308=CARTESIAN_POINT('Ctrl Pts',(38.3688154220767,264.631372142216,24.3127335164339)) ;
#100309=CARTESIAN_POINT('Ctrl Pts',(38.3937419849194,264.628574014862,24.2483163755689)) ;
#100310=CARTESIAN_POINT('Ctrl Pts',(38.4220471986119,264.625775887508,24.1852792627708)) ;
#100311=CARTESIAN_POINT('Ctrl Pts',(38.4535396282047,264.622977760155,24.1239862810453)) ;
#100312=CARTESIAN_POINT('Ctrl Pts',(38.4850805624662,264.620175323123,24.0625988958135)) ;
#100313=CARTESIAN_POINT('Ctrl Pts',(38.5198182578509,264.617372886091,24.0029614198518)) ;
#100314=CARTESIAN_POINT('Ctrl Pts',(38.5575171531634,264.614570449059,23.9454103343824)) ;
#100315=CARTESIAN_POINT('Ctrl Pts',(38.5627798025449,264.614179237502,23.9373763805533)) ;
#100316=CARTESIAN_POINT('Ctrl Pts',(38.5681000930982,264.613788025946,23.9293830327128)) ;
#100317=CARTESIAN_POINT('Ctrl Pts',(38.5734773222752,264.613396814389,23.9214311542105)) ;
#100318=CARTESIAN_POINT('Ctrl Pts',(38.6120240045259,264.610592413263,23.8644280911393)) ;
#100319=CARTESIAN_POINT('Ctrl Pts',(38.6536411680877,264.607788012137,23.8093498236701)) ;
#100320=CARTESIAN_POINT('Ctrl Pts',(38.6981100832999,264.60498361101,23.7565441071784)) ;
#100321=CARTESIAN_POINT('Ctrl Pts',(38.7436373142871,264.602112467938,23.7024816673664)) ;
#100322=CARTESIAN_POINT('Ctrl Pts',(38.7921535637017,264.599241324865,23.6508018123646)) ;
#100323=CARTESIAN_POINT('Ctrl Pts',(38.8433765377836,264.596370181792,23.6018468384303)) ;
#100324=CARTESIAN_POINT('Ctrl Pts',(38.8932818704625,264.593572894974,23.5541511646772)) ;
#100325=CARTESIAN_POINT('Ctrl Pts',(38.9457559699578,264.590775608155,23.5090422261409)) ;
#100326=CARTESIAN_POINT('Ctrl Pts',(39.0004980967225,264.587978321337,23.4668019506051)) ;
#100327=CARTESIAN_POINT('Ctrl Pts',(39.0552092963014,264.585182614877,23.4245855391925)) ;
#100328=CARTESIAN_POINT('Ctrl Pts',(39.1121855951858,264.582386908417,23.3852348717268)) ;
#100329=CARTESIAN_POINT('Ctrl Pts',(39.1710927569323,264.579591201957,23.3489919861002)) ;
#100330=CARTESIAN_POINT('Ctrl Pts',(39.2299863882496,264.576796137646,23.3127574251286)) ;
#100331=CARTESIAN_POINT('Ctrl Pts',(39.2908095864941,264.574001073334,23.279629483272)) ;
#100332=CARTESIAN_POINT('Ctrl Pts',(39.3532001618077,264.571206009022,23.2498062216747)) ;
#100333=CARTESIAN_POINT('Ctrl Pts',(39.4185466133079,264.568278523042,23.2185700244166)) ;
#100334=CARTESIAN_POINT('Ctrl Pts',(39.4856121449566,264.565351037063,23.1909597123105)) ;
#100335=CARTESIAN_POINT('Ctrl Pts',(39.5539551010565,264.562423551083,23.1671471481571)) ;
#100336=CARTESIAN_POINT('Ctrl Pts',(39.6192821921514,264.559625250363,23.1443853942555)) ;
#100337=CARTESIAN_POINT('Ctrl Pts',(39.6857758327279,264.556826949643,23.1250933516415)) ;
#100338=CARTESIAN_POINT('Ctrl Pts',(39.7530351849693,264.554028648923,23.1093698462599)) ;
#100339=CARTESIAN_POINT('Ctrl Pts',(39.8203378155972,264.551228547621,23.0936362235055)) ;
#100340=CARTESIAN_POINT('Ctrl Pts',(39.8884066590657,264.54842844632,23.0814757934472)) ;
#100341=CARTESIAN_POINT('Ctrl Pts',(39.9568325990537,264.545628345018,23.0729359191923)) ;
#100342=CARTESIAN_POINT('Ctrl Pts',(40.0253635085923,264.542823948191,23.0643829442514)) ;
#100343=CARTESIAN_POINT('Ctrl Pts',(40.0942521223562,264.540019551364,23.0594616370781)) ;
#100344=CARTESIAN_POINT('Ctrl Pts',(40.1630872342562,264.537215154537,23.0581673444979)) ;
#100345=CARTESIAN_POINT('Ctrl Pts',(40.1724061279648,264.536835495447,23.0579921232387)) ;
#100346=CARTESIAN_POINT('Ctrl Pts',(40.1817240472912,264.536455836357,23.0578832990001)) ;
#100347=CARTESIAN_POINT('Ctrl Pts',(40.1910399792807,264.536076177267,23.0578407872543)) ;
#100348=CARTESIAN_POINT('Ctrl Pts',(40.2598577696874,264.533271594782,23.0575267484216)) ;
#100349=CARTESIAN_POINT('Ctrl Pts',(40.328817304762,264.530467012297,23.0608344361905)) ;
#100350=CARTESIAN_POINT('Ctrl Pts',(40.3975079933341,264.527662429813,23.0677792401863)) ;
#100351=CARTESIAN_POINT('Ctrl Pts',(40.467828348868,264.52479130941,23.0748888076727)) ;
#100352=CARTESIAN_POINT('Ctrl Pts',(40.5378664243726,264.521920189007,23.0858103714212)) ;
#100353=CARTESIAN_POINT('Ctrl Pts',(40.6071804018321,264.519049068604,23.1005037540946)) ;
#100354=CARTESIAN_POINT('Ctrl Pts',(40.6747167858233,264.516251579597,23.1148203172286)) ;
#100355=CARTESIAN_POINT('Ctrl Pts',(40.7415652589116,264.513454090589,23.1327174456261)) ;
#100356=CARTESIAN_POINT('Ctrl Pts',(40.8073233679819,264.510656601582,23.1541056861881)) ;
#100357=CARTESIAN_POINT('Ctrl Pts',(40.8730444977572,264.507860685751,23.1754818990006)) ;
#100358=CARTESIAN_POINT('Ctrl Pts',(40.9376760178087,264.505064769921,23.2003451774765)) ;
#100359=CARTESIAN_POINT('Ctrl Pts',(41.000829537948,264.502268854091,23.2285559136498)) ;
#100360=CARTESIAN_POINT('Ctrl Pts',(41.0639687081095,264.499473573559,23.2567602396746)) ;
#100361=CARTESIAN_POINT('Ctrl Pts',(41.1256301007614,264.496678293028,23.2883103137473)) ;
#100362=CARTESIAN_POINT('Ctrl Pts',(41.1854458883187,264.493883012496,23.323018647395)) ;
#100363=CARTESIAN_POINT('Ctrl Pts',(41.2480865129882,264.490955723133,23.3593661033044)) ;
#100364=CARTESIAN_POINT('Ctrl Pts',(41.3087023701218,264.488028433771,23.3991772597833)) ;
#100365=CARTESIAN_POINT('Ctrl Pts',(41.3669026307358,264.485101144408,23.4421843454955)) ;
#100366=CARTESIAN_POINT('Ctrl Pts',(41.4225429371107,264.482302612662,23.483299752885)) ;
#100367=CARTESIAN_POINT('Ctrl Pts',(41.4759753345706,264.479504080915,23.5273354694665)) ;
#100368=CARTESIAN_POINT('Ctrl Pts',(41.5268921597548,264.476705549169,23.57401614389)) ;
#100369=CARTESIAN_POINT('Ctrl Pts',(41.5778418347219,264.473905211906,23.6207269350777)) ;
#100370=CARTESIAN_POINT('Ctrl Pts',(41.6262723664498,264.471104874643,23.6700857326611)) ;
#100371=CARTESIAN_POINT('Ctrl Pts',(41.6719139265479,264.46830453738,23.7217813318965)) ;
#100372=CARTESIAN_POINT('Ctrl Pts',(41.7176255853711,264.465499899211,23.773556327971)) ;
#100373=CARTESIAN_POINT('Ctrl Pts',(41.76053942759,264.462695261042,23.8276749028311)) ;
#100374=CARTESIAN_POINT('Ctrl Pts',(41.8004274053468,264.459890622873,23.8837947964993)) ;
#100375=CARTESIAN_POINT('Ctrl Pts',(41.8058085100117,264.459512261963,23.8913656747085)) ;
#100376=CARTESIAN_POINT('Ctrl Pts',(41.8111346129118,264.459133901054,23.8989729373091)) ;
#100377=CARTESIAN_POINT('Ctrl Pts',(41.8164052178499,264.458755540145,23.9066157092696)) ;
#100378=CARTESIAN_POINT('Ctrl Pts',(41.8558043111795,264.455927197487,23.9637473458282)) ;
#100379=CARTESIAN_POINT('Ctrl Pts',(41.8922413848146,264.453098854829,24.0230724888577)) ;
#100380=CARTESIAN_POINT('Ctrl Pts',(41.9254686504755,264.450270512171,24.0842556786478)) ;
#100381=CARTESIAN_POINT('Ctrl Pts',(41.958646693795,264.447446359375,24.1453482326363)) ;
#100382=CARTESIAN_POINT('Ctrl Pts',(41.9886241443276,264.444622206579,24.2082929534042)) ;
#100383=CARTESIAN_POINT('Ctrl Pts',(42.0151963518414,264.441798053783,24.2727253567599)) ;
#100384=CARTESIAN_POINT('Ctrl Pts',(42.0417338908785,264.438977585629,24.3370736958436)) ;
#100385=CARTESIAN_POINT('Ctrl Pts',(42.0648748369969,264.436157117475,24.4029054215471)) ;
#100386=CARTESIAN_POINT('Ctrl Pts',(42.0844611807787,264.433336649321,24.4698329836516)) ;
#100387=CARTESIAN_POINT('Ctrl Pts',(42.1040323458009,264.430518366936,24.5367086791402)) ;
#100388=CARTESIAN_POINT('Ctrl Pts',(42.1200542458913,264.42770008455,24.6046780688452)) ;
#100389=CARTESIAN_POINT('Ctrl Pts',(42.132418041646,264.424881802164,24.6733364900244)) ;
#100390=CARTESIAN_POINT('Ctrl Pts',(42.1447777802695,264.422064444587,24.7419723812117)) ;
#100391=CARTESIAN_POINT('Ctrl Pts',(42.1534817087956,264.41924708701,24.8112963876716)) ;
#100392=CARTESIAN_POINT('Ctrl Pts',(42.1584719621315,264.416429729432,24.8808930543848)) ;
#100393=CARTESIAN_POINT('Ctrl Pts',(42.161847349748,264.414524079912,24.927967964448)) ;
#100394=CARTESIAN_POINT('Ctrl Pts',(42.1635247492932,264.412618430391,24.975167391973)) ;
#100395=CARTESIAN_POINT('Ctrl Pts',(42.1634997239518,264.41071278087,25.0223615166147)) ;
#100396=CARTESIAN_POINT('',(42.1634998081267,263.910712780839,25.0204523075086)) ;
#100397=CARTESIAN_POINT('Ctrl Pts',(42.1634997239514,264.410712780843,25.0223615172765)) ;
#100398=CARTESIAN_POINT('Ctrl Pts',(42.163458777492,264.407594759394,25.0995804871246)) ;
#100399=CARTESIAN_POINT('Ctrl Pts',(42.1588584816758,264.404476737946,25.176643865133)) ;
#100400=CARTESIAN_POINT('Ctrl Pts',(42.1497783422879,264.401358716497,25.2530457542185)) ;
#100401=CARTESIAN_POINT('Ctrl Pts',(42.1406617510449,264.398228177876,25.329754355621)) ;
#100402=CARTESIAN_POINT('Ctrl Pts',(42.1270294057865,264.395097639255,25.4057958914338)) ;
#100403=CARTESIAN_POINT('Ctrl Pts',(42.1090116562539,264.391967100634,25.4806750499541)) ;
#100404=CARTESIAN_POINT('Ctrl Pts',(42.0909101969885,264.388822017658,25.555902094005)) ;
#100405=CARTESIAN_POINT('Ctrl Pts',(42.0683826202559,264.385676934682,25.6299556886429)) ;
#100406=CARTESIAN_POINT('Ctrl Pts',(42.0416093908855,264.382531851706,25.7023541910313)) ;
#100407=CARTESIAN_POINT('Ctrl Pts',(42.0384967163878,264.382166202145,25.7107712918952)) ;
#100408=CARTESIAN_POINT('Ctrl Pts',(42.0353267074247,264.381800552583,25.7191660468239)) ;
#100409=CARTESIAN_POINT('Ctrl Pts',(42.0320996884114,264.381434903022,25.727537719247)) ;
#100410=CARTESIAN_POINT('Ctrl Pts',(42.0073503843503,264.378630589774,25.7917434352487)) ;
#100411=CARTESIAN_POINT('Ctrl Pts',(41.9791767836945,264.375826276526,25.8547637148073)) ;
#100412=CARTESIAN_POINT('Ctrl Pts',(41.9477138619951,264.373021963277,25.9162105639722)) ;
#100413=CARTESIAN_POINT('Ctrl Pts',(41.9155010215255,264.37015080922,25.9791219988485)) ;
#100414=CARTESIAN_POINT('Ctrl Pts',(41.8798401431771,264.367279655162,26.0403835214419)) ;
#100415=CARTESIAN_POINT('Ctrl Pts',(41.8409293882998,264.364408501105,26.0995981336555)) ;
#100416=CARTESIAN_POINT('Ctrl Pts',(41.8030208276166,264.36161129714,26.157287600938)) ;
#100417=CARTESIAN_POINT('Ctrl Pts',(41.7620280728643,264.358814093176,26.2130338974303)) ;
#100418=CARTESIAN_POINT('Ctrl Pts',(41.7181808066942,264.356016889211,26.2664947442704)) ;
#100419=CARTESIAN_POINT('Ctrl Pts',(41.6743582796633,264.353221263461,26.3199254278767)) ;
#100420=CARTESIAN_POINT('Ctrl Pts',(41.6276847458526,264.350425637712,26.3710728446154)) ;
#100421=CARTESIAN_POINT('Ctrl Pts',(41.5784314916249,264.347630011962,26.4196260586651)) ;
#100422=CARTESIAN_POINT('Ctrl Pts',(41.529189509994,264.344835026048,26.4681681603364)) ;
#100423=CARTESIAN_POINT('Ctrl Pts',(41.4773693277752,264.342040040133,26.5141168967294)) ;
#100424=CARTESIAN_POINT('Ctrl Pts',(41.4232793512456,264.339245054219,26.5571979033983)) ;
#100425=CARTESIAN_POINT('Ctrl Pts',(41.3666236239985,264.336317488525,26.6023224517891)) ;
#100426=CARTESIAN_POINT('Ctrl Pts',(41.3074778346146,264.333389922832,26.6443000433091)) ;
#100427=CARTESIAN_POINT('Ctrl Pts',(41.246233771239,264.330462357139,26.6828639469354)) ;
#100428=CARTESIAN_POINT('Ctrl Pts',(41.1876954001309,264.327664127931,26.7197241416617)) ;
#100429=CARTESIAN_POINT('Ctrl Pts',(41.1272407212263,264.324865898722,26.7534657207546)) ;
#100430=CARTESIAN_POINT('Ctrl Pts',(41.0652380983901,264.322067669514,26.7839023368564)) ;
#100431=CARTESIAN_POINT('Ctrl Pts',(41.0031955236829,264.319267637244,26.814358565028)) ;
#100432=CARTESIAN_POINT('Ctrl Pts',(40.9396034679074,264.316467604975,26.8415054008056)) ;
#100433=CARTESIAN_POINT('Ctrl Pts',(40.8748499230125,264.313667572706,26.8652047844642)) ;
#100434=CARTESIAN_POINT('Ctrl Pts',(40.8099969463639,264.310863240871,26.8889405595093)) ;
#100435=CARTESIAN_POINT('Ctrl Pts',(40.7439793882218,264.308058909036,26.9092181818454)) ;
#100436=CARTESIAN_POINT('Ctrl Pts',(40.6771989624199,264.305254577201,26.9259498089059)) ;
#100437=CARTESIAN_POINT('Ctrl Pts',(40.6681474332564,264.304874473434,26.9282176412606)) ;
#100438=CARTESIAN_POINT('Ctrl Pts',(40.659081900542,264.304494369668,26.9304204057263)) ;
#100439=CARTESIAN_POINT('Ctrl Pts',(40.650003373869,264.304114265901,26.9325579566016)) ;
#100440=CARTESIAN_POINT('Ctrl Pts',(40.5830244210172,264.301309961504,26.9483282378873)) ;
#100441=CARTESIAN_POINT('Ctrl Pts',(40.5150933063956,264.298505657107,26.9606021865817)) ;
#100442=CARTESIAN_POINT('Ctrl Pts',(40.4466065577867,264.29570135271,26.9692724619795)) ;
#100443=CARTESIAN_POINT('Ctrl Pts',(40.3764871791172,264.292830197546,26.9781494248393)) ;
#100444=CARTESIAN_POINT('Ctrl Pts',(40.3057858146515,264.289959042382,26.9832484865257)) ;
#100445=CARTESIAN_POINT('Ctrl Pts',(40.2349420653057,264.287087887218,26.9845094078303)) ;
#100446=CARTESIAN_POINT('Ctrl Pts',(40.16592320119,264.284290690995,26.9857378486877)) ;
#100447=CARTESIAN_POINT('Ctrl Pts',(40.0967697192689,264.281493494772,26.9833234985888)) ;
#100448=CARTESIAN_POINT('Ctrl Pts',(40.0278938043149,264.278696298549,26.9772630082118)) ;
#100449=CARTESIAN_POINT('Ctrl Pts',(39.9590567393324,264.275900680105,26.9712059362994)) ;
#100450=CARTESIAN_POINT('Ctrl Pts',(39.8904974152564,264.273105061661,26.9615068481148)) ;
#100451=CARTESIAN_POINT('Ctrl Pts',(39.8226255951793,264.270309443217,26.9482144269451)) ;
#100452=CARTESIAN_POINT('Ctrl Pts',(39.7547692980579,264.267514464159,26.9349250458835)) ;
#100453=CARTESIAN_POINT('Ctrl Pts',(39.6876006707138,264.264719485101,26.9180440580319)) ;
#100454=CARTESIAN_POINT('Ctrl Pts',(39.6215202082828,264.261924506042,26.897671424934)) ;
#100455=CARTESIAN_POINT('Ctrl Pts',(39.5523048830281,264.258996932937,26.876332312369)) ;
#100456=CARTESIAN_POINT('Ctrl Pts',(39.4842841046609,264.256069359832,26.8511621497015)) ;
#100457=CARTESIAN_POINT('Ctrl Pts',(39.4178990926936,264.253141786726,26.8223340638823)) ;
#100458=CARTESIAN_POINT('Ctrl Pts',(39.3544471827243,264.250343563158,26.7947796950303)) ;
#100459=CARTESIAN_POINT('Ctrl Pts',(39.2924899691217,264.247545339589,26.7638841088208)) ;
#100460=CARTESIAN_POINT('Ctrl Pts',(39.2323890731672,264.24474711602,26.7298464171897)) ;
#100461=CARTESIAN_POINT('Ctrl Pts',(39.1722494414693,264.241947088962,26.6957867878608)) ;
#100462=CARTESIAN_POINT('Ctrl Pts',(39.1139689189766,264.239147061905,26.6585812848545)) ;
#100463=CARTESIAN_POINT('Ctrl Pts',(39.0578803190547,264.236347034848,26.6184724604218)) ;
#100464=CARTESIAN_POINT('Ctrl Pts',(39.0017055797137,264.233542707581,26.5783020378954)) ;
#100465=CARTESIAN_POINT('Ctrl Pts',(38.9477298566808,264.230738380315,26.535219704408)) ;
#100466=CARTESIAN_POINT('Ctrl Pts',(38.8962522312928,264.227934053049,26.489507663213)) ;
#100467=CARTESIAN_POINT('Ctrl Pts',(38.8892741663483,264.227553911625,26.4833111537625)) ;
#100468=CARTESIAN_POINT('Ctrl Pts',(38.882341947018,264.227173770202,26.4770663760187)) ;
#100469=CARTESIAN_POINT('Ctrl Pts',(38.8754562631737,264.226793628778,26.4707740817777)) ;
#100470=CARTESIAN_POINT('Ctrl Pts',(38.8246612808289,264.22398936455,26.424356473576)) ;
#100471=CARTESIAN_POINT('Ctrl Pts',(38.7762165292526,264.221185100322,26.3751808753811)) ;
#100472=CARTESIAN_POINT('Ctrl Pts',(38.7304342718421,264.218380836093,26.3235141926557)) ;
#100473=CARTESIAN_POINT('Ctrl Pts',(38.6835598748704,264.215509675908,26.2706149969134)) ;
#100474=CARTESIAN_POINT('Ctrl Pts',(38.6394770748674,264.212638515723,26.2151046178442)) ;
#100475=CARTESIAN_POINT('Ctrl Pts',(38.5984835450502,264.209767355539,26.1573121104862)) ;
#100476=CARTESIAN_POINT('Ctrl Pts',(38.5585466517975,264.206970201492,26.1010092449497)) ;
#100477=CARTESIAN_POINT('Ctrl Pts',(38.5215419890435,264.204173047445,26.0425409069009)) ;
#100478=CARTESIAN_POINT('Ctrl Pts',(38.487704774341,264.201375893399,25.9822455800819)) ;
#100479=CARTESIAN_POINT('Ctrl Pts',(38.4538866535994,264.198580317754,25.9219842772399)) ;
#100480=CARTESIAN_POINT('Ctrl Pts',(38.4232326720322,264.195784742111,25.8598984558136)) ;
#100481=CARTESIAN_POINT('Ctrl Pts',(38.3959337131029,264.192989166466,25.796353944432)) ;
#100482=CARTESIAN_POINT('Ctrl Pts',(38.3686410031823,264.190194230758,25.7328239790339)) ;
#100483=CARTESIAN_POINT('Ctrl Pts',(38.3447019826041,264.18739929505,25.6678364346535)) ;
#100484=CARTESIAN_POINT('Ctrl Pts',(38.3242599624995,264.184604359341,25.6017784055398)) ;
#100485=CARTESIAN_POINT('Ctrl Pts',(38.3028475401916,264.181676745368,25.5325845387411)) ;
#100486=CARTESIAN_POINT('Ctrl Pts',(38.2852726126217,264.178749131394,25.4622165629685)) ;
#100487=CARTESIAN_POINT('Ctrl Pts',(38.2716410456622,264.17582151742,25.3911365049494)) ;
#100488=CARTESIAN_POINT('Ctrl Pts',(38.2586121526955,264.173023338074,25.3231990131888)) ;
#100489=CARTESIAN_POINT('Ctrl Pts',(38.2491852999413,264.170225158729,25.254611589662)) ;
#100490=CARTESIAN_POINT('Ctrl Pts',(38.2433999949789,264.167426979383,25.1857851432934)) ;
#100491=CARTESIAN_POINT('Ctrl Pts',(38.2376109617994,264.164626996811,25.1169143431799)) ;
#100492=CARTESIAN_POINT('Ctrl Pts',(38.2354681618351,264.161827014238,25.0478047004715)) ;
#100493=CARTESIAN_POINT('Ctrl Pts',(38.2369589830322,264.159027031665,24.9788678324192)) ;
#100494=CARTESIAN_POINT('Ctrl Pts',(38.2384520937988,264.156222748942,24.9098250926849)) ;
#100495=CARTESIAN_POINT('Ctrl Pts',(38.2435899192609,264.153418466219,24.8409561416085)) ;
#100496=CARTESIAN_POINT('Ctrl Pts',(38.2523080800396,264.150614183497,24.7726671012301)) ;
#100497=CARTESIAN_POINT('Ctrl Pts',(38.2534906871367,264.150233786216,24.7634037822969)) ;
#100498=CARTESIAN_POINT('Ctrl Pts',(38.2547390979433,264.149853388936,24.7541511165292)) ;
#100499=CARTESIAN_POINT('Ctrl Pts',(38.2560530801867,264.149472991656,24.7449100996315)) ;
#100500=CARTESIAN_POINT('Ctrl Pts',(38.2657397501837,264.146668704961,24.676785373007)) ;
#100501=CARTESIAN_POINT('Ctrl Pts',(38.2790294654451,264.143864418266,24.6090461664029)) ;
#100502=CARTESIAN_POINT('Ctrl Pts',(38.2958779051084,264.141060131571,24.5421008763572)) ;
#100503=CARTESIAN_POINT('Ctrl Pts',(38.3131281106275,264.138188974194,24.4735592170166)) ;
#100504=CARTESIAN_POINT('Ctrl Pts',(38.3341089620186,264.135317816818,24.4058503462897)) ;
#100505=CARTESIAN_POINT('Ctrl Pts',(38.3587165892024,264.132446659441,24.3394056486588)) ;
#100506=CARTESIAN_POINT('Ctrl Pts',(38.3826901607964,264.12964948211,24.2746730068728)) ;
#100507=CARTESIAN_POINT('Ctrl Pts',(38.4101056754069,264.126852304779,24.2111406621024)) ;
#100508=CARTESIAN_POINT('Ctrl Pts',(38.4408162530818,264.124055127449,24.1491937503526)) ;
#100509=CARTESIAN_POINT('Ctrl Pts',(38.4715095038536,264.121259528285,24.0872817890406)) ;
#100510=CARTESIAN_POINT('Ctrl Pts',(38.5054939122858,264.118463929121,24.026953921516)) ;
#100511=CARTESIAN_POINT('Ctrl Pts',(38.542575014903,264.115668329957,23.9685740926633)) ;
#100512=CARTESIAN_POINT('Ctrl Pts',(38.5796476319375,264.112873370534,23.9102076233611)) ;
#100513=CARTESIAN_POINT('Ctrl Pts',(38.6198152742216,264.110078411111,23.8537887184565)) ;
#100514=CARTESIAN_POINT('Ctrl Pts',(38.6628390888999,264.107283451688,23.7996540293043)) ;
#100515=CARTESIAN_POINT('Ctrl Pts',(38.7079045557083,264.104355860258,23.7429504325776)) ;
#100516=CARTESIAN_POINT('Ctrl Pts',(38.7561036911565,264.101428268829,23.6887537206051)) ;
#100517=CARTESIAN_POINT('Ctrl Pts',(38.8071146606288,264.098500677399,23.6374118634335)) ;
#100518=CARTESIAN_POINT('Ctrl Pts',(38.8558711435674,264.095702474129,23.5883391167457)) ;
#100519=CARTESIAN_POINT('Ctrl Pts',(38.9071957379641,264.092904270859,23.541874496539)) ;
#100520=CARTESIAN_POINT('Ctrl Pts',(38.9607713858759,264.090106067589,23.498282362439)) ;
#100521=CARTESIAN_POINT('Ctrl Pts',(39.0143815601378,264.087306061042,23.4546621357755)) ;
#100522=CARTESIAN_POINT('Ctrl Pts',(39.0702452814918,264.084506054495,23.4139183662745)) ;
#100523=CARTESIAN_POINT('Ctrl Pts',(39.1280155143677,264.081706047947,23.3762727720397)) ;
#100524=CARTESIAN_POINT('Ctrl Pts',(39.1858744666936,264.078901741348,23.3385693643558)) ;
#100525=CARTESIAN_POINT('Ctrl Pts',(39.2456453492233,264.076097434748,23.3039738648127)) ;
#100526=CARTESIAN_POINT('Ctrl Pts',(39.3069564703197,264.073293128148,23.2726621425105)) ;
#100527=CARTESIAN_POINT('Ctrl Pts',(39.3152701248978,264.072912870277,23.2684163411158)) ;
#100528=CARTESIAN_POINT('Ctrl Pts',(39.3236120708399,264.072532612405,23.2642308447827)) ;
#100529=CARTESIAN_POINT('Ctrl Pts',(39.3319813559531,264.072152354534,23.2601060228175)) ;
#100530=CARTESIAN_POINT('Ctrl Pts',(39.3937022339776,264.069348070849,23.2296867420853)) ;
#100531=CARTESIAN_POINT('Ctrl Pts',(39.4571366665362,264.066543787163,23.2024603023848)) ;
#100532=CARTESIAN_POINT('Ctrl Pts',(39.5219224013884,264.063739503478,23.1786204167508)) ;
#100533=CARTESIAN_POINT('Ctrl Pts',(39.5882530889276,264.060868345726,23.1542120186896)) ;
#100534=CARTESIAN_POINT('Ctrl Pts',(39.6559999355778,264.057997187973,23.1333540793622)) ;
#100535=CARTESIAN_POINT('Ctrl Pts',(39.7247481213259,264.05512603022,23.1162040999102)) ;
#100536=CARTESIAN_POINT('Ctrl Pts',(39.7917248172262,264.0523288559,23.0994960377853)) ;
#100537=CARTESIAN_POINT('Ctrl Pts',(39.8596513637146,264.049531681581,23.0863072672656)) ;
#100538=CARTESIAN_POINT('Ctrl Pts',(39.9281268794345,264.046734507261,23.0767336891999)) ;
#100539=CARTESIAN_POINT('Ctrl Pts',(39.9965637614437,264.0439389111,23.0671655125224)) ;
#100540=CARTESIAN_POINT('Ctrl Pts',(40.0655485162028,264.041143314939,23.0612085479421)) ;
#100541=CARTESIAN_POINT('Ctrl Pts',(40.1346709276571,264.038347718779,23.0589074506375)) ;
#100542=CARTESIAN_POINT('Ctrl Pts',(40.203777521568,264.035552762344,23.0566068799017)) ;
#100543=CARTESIAN_POINT('Ctrl Pts',(40.2730212226455,264.03275780591,23.057960530788)) ;
#100544=CARTESIAN_POINT('Ctrl Pts',(40.3419893209184,264.029962849476,23.0629610091306)) ;
#100545=CARTESIAN_POINT('Ctrl Pts',(40.414230380419,264.027035255138,23.0681987909823)) ;
#100546=CARTESIAN_POINT('Ctrl Pts',(40.486168446313,264.024107660799,23.0774381490376)) ;
#100547=CARTESIAN_POINT('Ctrl Pts',(40.5573346615202,264.02118006646,23.0906095444816)) ;
#100548=CARTESIAN_POINT('Ctrl Pts',(40.625355468153,264.018381866109,23.1031987898135)) ;
#100549=CARTESIAN_POINT('Ctrl Pts',(40.6926707318042,264.015583665757,23.1193796467942)) ;
#100550=CARTESIAN_POINT('Ctrl Pts',(40.7588833384476,264.012785465405,23.1390393698456)) ;
#100551=CARTESIAN_POINT('Ctrl Pts',(40.8251386159097,264.009985461749,23.1587117626365)) ;
#100552=CARTESIAN_POINT('Ctrl Pts',(40.8902893632423,264.007185458093,23.1818673202467)) ;
#100553=CARTESIAN_POINT('Ctrl Pts',(40.953956774569,264.004385454437,23.2083444937256)) ;
#100554=CARTESIAN_POINT('Ctrl Pts',(41.0177219632648,264.001581150669,23.2348623295827)) ;
#100555=CARTESIAN_POINT('Ctrl Pts',(41.0799988342206,263.998776846901,23.2647117450629)) ;
#100556=CARTESIAN_POINT('Ctrl Pts',(41.1404325395613,263.995972543133,23.2976849736121)) ;
#100557=CARTESIAN_POINT('Ctrl Pts',(41.1486276010531,263.995592267892,23.3021562803774)) ;
#100558=CARTESIAN_POINT('Ctrl Pts',(41.1567888136466,263.995211992652,23.306684964509)) ;
#100559=CARTESIAN_POINT('Ctrl Pts',(41.1649153352637,263.994831717412,23.3112704478627)) ;
#100560=CARTESIAN_POINT('Ctrl Pts',(41.2248431157155,263.992027436295,23.3450853877143)) ;
#100561=CARTESIAN_POINT('Ctrl Pts',(41.2831005702371,263.989223155179,23.3821159857416)) ;
#100562=CARTESIAN_POINT('Ctrl Pts',(41.3393234378276,263.986418874063,23.4221723347697)) ;
#100563=CARTESIAN_POINT('Ctrl Pts',(41.3968871176164,263.983547715989,23.4631839542011)) ;
#100564=CARTESIAN_POINT('Ctrl Pts',(41.4523174277952,263.980676557915,23.5073673238773)) ;
#100565=CARTESIAN_POINT('Ctrl Pts',(41.5052503649183,263.977805399841,23.5544687031812)) ;
#100566=CARTESIAN_POINT('Ctrl Pts',(41.5568192802853,263.975008228254,23.6003563333603)) ;
#100567=CARTESIAN_POINT('Ctrl Pts',(41.6060175953642,263.972211056668,23.6490130484477)) ;
#100568=CARTESIAN_POINT('Ctrl Pts',(41.6525400386672,263.969413885081,23.7001618799116)) ;
#100569=CARTESIAN_POINT('Ctrl Pts',(41.6990362332188,263.966618291706,23.7512818523374)) ;
#100570=CARTESIAN_POINT('Ctrl Pts',(41.7428592247573,263.963822698331,23.8048907908515)) ;
#100571=CARTESIAN_POINT('Ctrl Pts',(41.7837407967197,263.961027104956,23.8606751183484)) ;
#100572=CARTESIAN_POINT('Ctrl Pts',(41.8246130128812,263.958232151356,23.9164466795294)) ;
#100573=CARTESIAN_POINT('Ctrl Pts',(41.8625448586599,263.955437197757,23.9743922477505)) ;
#100574=CARTESIAN_POINT('Ctrl Pts',(41.8973096939531,263.952642244157,24.0341668333026)) ;
#100575=CARTESIAN_POINT('Ctrl Pts',(41.9337244047851,263.949714647168,24.0967782114271)) ;
#100576=CARTESIAN_POINT('Ctrl Pts',(41.9666636898901,263.946787050179,24.1613960540462)) ;
#100577=CARTESIAN_POINT('Ctrl Pts',(41.995920563786,263.94385945319,24.2275939558348)) ;
#100578=CARTESIAN_POINT('Ctrl Pts',(42.0238842861241,263.941061255761,24.2908659154972)) ;
#100579=CARTESIAN_POINT('Ctrl Pts',(42.0484841324827,263.938263058332,24.3555807041393)) ;
#100580=CARTESIAN_POINT('Ctrl Pts',(42.069589258488,263.935464860903,24.4213467986874)) ;
#100581=CARTESIAN_POINT('Ctrl Pts',(42.0907079855291,263.932664860197,24.4871552756885)) ;
#100582=CARTESIAN_POINT('Ctrl Pts',(42.1083273859935,263.929864859491,24.5540159359917)) ;
#100583=CARTESIAN_POINT('Ctrl Pts',(42.1223672427004,263.927064858785,24.621524853099)) ;
#100584=CARTESIAN_POINT('Ctrl Pts',(42.1364286610765,263.924260557987,24.6891374468305)) ;
#100585=CARTESIAN_POINT('Ctrl Pts',(42.1468994981384,263.921456257188,24.7573998024067)) ;
#100586=CARTESIAN_POINT('Ctrl Pts',(42.1537512147579,263.918651956389,24.8259017138642)) ;
#100587=CARTESIAN_POINT('Ctrl Pts',(42.1546803780079,263.918271664356,24.8351912776649)) ;
#100588=CARTESIAN_POINT('Ctrl Pts',(42.1555430635202,263.917891372322,24.8444852468158)) ;
#100589=CARTESIAN_POINT('Ctrl Pts',(42.1563392738469,263.917511080289,24.8537825997396)) ;
#100590=CARTESIAN_POINT('Ctrl Pts',(42.1610837646848,263.915244980483,24.9091840486851)) ;
#100591=CARTESIAN_POINT('Ctrl Pts',(42.163475200471,263.912978880676,24.9647897749953)) ;
#100592=CARTESIAN_POINT('Ctrl Pts',(42.1634998081263,263.91071278087,25.0204523067486)) ;
#100593=CARTESIAN_POINT('',(42.1634999347757,263.410712780838,25.0218264420184)) ;
#100594=CARTESIAN_POINT('Ctrl Pts',(42.1634998081267,263.910712780839,25.0204523075086)) ;
#100595=CARTESIAN_POINT('Ctrl Pts',(42.1635299115909,263.907940573848,25.0885464220032)) ;
#100596=CARTESIAN_POINT('Ctrl Pts',(42.1600135022032,263.905168366856,25.1567718338227)) ;
#100597=CARTESIAN_POINT('Ctrl Pts',(42.1529358967757,263.902396159865,25.2247254395744)) ;
#100598=CARTESIAN_POINT('Ctrl Pts',(42.145868575163,263.899627980912,25.2925803082184)) ;
#100599=CARTESIAN_POINT('Ctrl Pts',(42.135250383065,263.896859801958,25.3601636613063)) ;
#100600=CARTESIAN_POINT('Ctrl Pts',(42.1211186552297,263.894091623005,25.4270731778424)) ;
#100601=CARTESIAN_POINT('Ctrl Pts',(42.1069981500108,263.891325642382,25.4939295586369)) ;
#100602=CARTESIAN_POINT('Ctrl Pts',(42.0893697436254,263.888559661759,25.5601126766334)) ;
#100603=CARTESIAN_POINT('Ctrl Pts',(42.0683222959035,263.885793681136,25.6252276614734)) ;
#100604=CARTESIAN_POINT('Ctrl Pts',(42.0472840797745,263.883028913697,25.6903140863168)) ;
#100605=CARTESIAN_POINT('Ctrl Pts',(42.0228299507088,263.880264146257,25.7543328324265)) ;
#100606=CARTESIAN_POINT('Ctrl Pts',(41.9950988482286,263.877499378817,25.8169033845355)) ;
#100607=CARTESIAN_POINT('Ctrl Pts',(41.967370049988,263.874734841108,25.8794687375166)) ;
#100608=CARTESIAN_POINT('Ctrl Pts',(41.936365023349,263.871970303399,25.9405856794601)) ;
#100609=CARTESIAN_POINT('Ctrl Pts',(41.9022703963241,263.86920576569,25.999894688103)) ;
#100610=CARTESIAN_POINT('Ctrl Pts',(41.8681453554388,263.866438761896,26.0592566029093)) ;
#100611=CARTESIAN_POINT('Ctrl Pts',(41.8309254621913,263.863671758102,26.1168069310684)) ;
#100612=CARTESIAN_POINT('Ctrl Pts',(41.7908421858289,263.860904754307,26.1722127754519)) ;
#100613=CARTESIAN_POINT('Ctrl Pts',(41.7507389843784,263.858136375057,26.2276461616541)) ;
#100614=CARTESIAN_POINT('Ctrl Pts',(41.7077698807821,263.855367995806,26.2809325532818)) ;
#100615=CARTESIAN_POINT('Ctrl Pts',(41.66220660755,263.852599616555,26.3317722071689)) ;
#100616=CARTESIAN_POINT('Ctrl Pts',(41.6165695611983,263.849826754923,26.3826941773516)) ;
#100617=CARTESIAN_POINT('Ctrl Pts',(41.5683303152164,263.847053893291,26.4311611497577)) ;
#100618=CARTESIAN_POINT('Ctrl Pts',(41.5177966623674,263.844281031659,26.476911016329)) ;
#100619=CARTESIAN_POINT('Ctrl Pts',(41.4929471980248,263.842917502162,26.4994080972632)) ;
#100620=CARTESIAN_POINT('Ctrl Pts',(41.4675434202115,263.841553972664,26.5212487856042)) ;
#100621=CARTESIAN_POINT('Ctrl Pts',(41.4416245545341,263.840190443167,26.5424057177507)) ;
#100622=CARTESIAN_POINT('Ctrl Pts',(41.3883188809768,263.837386159247,26.585917827135)) ;
#100623=CARTESIAN_POINT('Ctrl Pts',(41.3326259359026,263.834581875326,26.6267038710564)) ;
#100624=CARTESIAN_POINT('Ctrl Pts',(41.274855170085,263.831777591406,26.6644936799248)) ;
#100625=CARTESIAN_POINT('Ctrl Pts',(41.215706743906,263.828906433682,26.7031846629598)) ;
#100626=CARTESIAN_POINT('Ctrl Pts',(41.1543804641331,263.826035275959,26.7387342754357)) ;
#100627=CARTESIAN_POINT('Ctrl Pts',(41.0912451427048,263.823164118236,26.7708958193837)) ;
#100628=CARTESIAN_POINT('Ctrl Pts',(41.0297366771451,263.820366943818,26.8022286323562)) ;
#100629=CARTESIAN_POINT('Ctrl Pts',(40.966511742001,263.817569769401,26.8303456470779)) ;
#100630=CARTESIAN_POINT('Ctrl Pts',(40.9019394111395,263.814772594983,26.8550633225752)) ;
#100631=CARTESIAN_POINT('Ctrl Pts',(40.8374035129998,263.811976998775,26.8797670519724)) ;
#100632=CARTESIAN_POINT('Ctrl Pts',(40.7715221821602,263.809181402567,26.9010750743841)) ;
#100633=CARTESIAN_POINT('Ctrl Pts',(40.7046851052687,263.80638580636,26.9188516857302)) ;
#100634=CARTESIAN_POINT('Ctrl Pts',(40.6378633241782,263.80359084993,26.9366242288627)) ;
#100635=CARTESIAN_POINT('Ctrl Pts',(40.5700867023821,263.8007958935,26.9508668411144)) ;
#100636=CARTESIAN_POINT('Ctrl Pts',(40.5017590541382,263.79800093707,26.9614939758012)) ;
#100637=CARTESIAN_POINT('Ctrl Pts',(40.430188839982,263.795073342818,26.9726254331973)) ;
#100638=CARTESIAN_POINT('Ctrl Pts',(40.3580145641661,263.792145748566,26.9797895834629)) ;
#100639=CARTESIAN_POINT('Ctrl Pts',(40.2857087180477,263.789218154314,26.9829488164491)) ;
#100640=CARTESIAN_POINT('Ctrl Pts',(40.2165986511779,263.786419954093,26.9859684174171)) ;
#100641=CARTESIAN_POINT('Ctrl Pts',(40.1473689089545,263.783621753873,26.9853297205025)) ;
#100642=CARTESIAN_POINT('Ctrl Pts',(40.0784317851542,263.780823553653,26.9810533404597)) ;
#100643=CARTESIAN_POINT('Ctrl Pts',(40.009450235794,263.778023550172,26.976774204564)) ;
#100644=CARTESIAN_POINT('Ctrl Pts',(39.9407621639637,263.775223546692,26.9688527759084)) ;
#100645=CARTESIAN_POINT('Ctrl Pts',(39.8727729916271,263.772423543211,26.9573613387328)) ;
#100646=CARTESIAN_POINT('Ctrl Pts',(39.8046794062305,263.769619239678,26.9458522538042)) ;
#100647=CARTESIAN_POINT('Ctrl Pts',(39.7372873353663,263.766814936146,26.9307623320496)) ;
#100648=CARTESIAN_POINT('Ctrl Pts',(39.6709892427341,263.764010632614,26.9122142773108)) ;
#100649=CARTESIAN_POINT('Ctrl Pts',(39.6619989385297,263.763630357091,26.9096990819577)) ;
#100650=CARTESIAN_POINT('Ctrl Pts',(39.6530287225328,263.763250081568,26.9071203697549)) ;
#100651=CARTESIAN_POINT('Ctrl Pts',(39.6440795452144,263.762869806046,26.904478514811)) ;
#100652=CARTESIAN_POINT('Ctrl Pts',(39.5780851337236,263.760065519301,26.8849965383051)) ;
#100653=CARTESIAN_POINT('Ctrl Pts',(39.5129956509329,263.757261232556,26.8620057637291)) ;
#100654=CARTESIAN_POINT('Ctrl Pts',(39.4492087201761,263.754456945811,26.8356093790058)) ;
#100655=CARTESIAN_POINT('Ctrl Pts',(39.3839007352826,263.75158578844,26.8085835498226)) ;
#100656=CARTESIAN_POINT('Ctrl Pts',(39.3199587410339,263.74871463107,26.7779876613632)) ;
#100657=CARTESIAN_POINT('Ctrl Pts',(39.2577944526421,263.7458434737,26.7439871588573)) ;
#100658=CARTESIAN_POINT('Ctrl Pts',(39.1972319277987,263.743046296348,26.710862734353)) ;
#100659=CARTESIAN_POINT('Ctrl Pts',(39.1383570555545,263.740249118996,26.6745072863799)) ;
#100660=CARTESIAN_POINT('Ctrl Pts',(39.08152954437,263.737451941645,26.635122094049)) ;
#100661=CARTESIAN_POINT('Ctrl Pts',(39.0247340954781,263.734656342471,26.5957591229898)) ;
#100662=CARTESIAN_POINT('Ctrl Pts',(38.9699841151777,263.731860743297,26.5533700769759)) ;
#100663=CARTESIAN_POINT('Ctrl Pts',(38.9176114321015,263.729065144123,26.5082002347826)) ;
#100664=CARTESIAN_POINT('Ctrl Pts',(38.8652507341125,263.726270184701,26.4630407293614)) ;
#100665=CARTESIAN_POINT('Ctrl Pts',(38.8152666216021,263.723475225279,26.4151020100986)) ;
#100666=CARTESIAN_POINT('Ctrl Pts',(38.7679574698095,263.720680265856,26.3646693085443)) ;
#100667=CARTESIAN_POINT('Ctrl Pts',(38.7184033097922,263.717752674445,26.3118433738525)) ;
#100668=CARTESIAN_POINT('Ctrl Pts',(38.6717847350701,263.714825083034,26.2562812576785)) ;
#100669=CARTESIAN_POINT('Ctrl Pts',(38.6283992627555,263.711897491623,26.1983519373125)) ;
#100670=CARTESIAN_POINT('Ctrl Pts',(38.5869312597987,263.709099288381,26.1429828678969)) ;
#100671=CARTESIAN_POINT('Ctrl Pts',(38.5484168377012,263.706301085138,26.0854518825699)) ;
#100672=CARTESIAN_POINT('Ctrl Pts',(38.5130714843996,263.703502881896,26.0261110845869)) ;
#100673=CARTESIAN_POINT('Ctrl Pts',(38.4777033532163,263.700702875386,25.9667320451507)) ;
#100674=CARTESIAN_POINT('Ctrl Pts',(38.4455085820263,263.697902868876,25.9055413029229)) ;
#100675=CARTESIAN_POINT('Ctrl Pts',(38.4166561141778,263.695102862366,25.8429144251477)) ;
#100676=CARTESIAN_POINT('Ctrl Pts',(38.3877593368753,263.692298555816,25.7801913697152)) ;
#100677=CARTESIAN_POINT('Ctrl Pts',(38.3622152797791,263.689494249266,25.7160282316914)) ;
#100678=CARTESIAN_POINT('Ctrl Pts',(38.34014394139,263.686689942716,25.6508183111907)) ;
#100679=CARTESIAN_POINT('Ctrl Pts',(38.3371511154177,263.686309684785,25.641975986349)) ;
#100680=CARTESIAN_POINT('Ctrl Pts',(38.3342220651648,263.685929426854,25.6331144322903)) ;
#100681=CARTESIAN_POINT('Ctrl Pts',(38.3313570176715,263.685549168922,25.624234644762)) ;
#100682=CARTESIAN_POINT('Ctrl Pts',(38.3102283420653,263.682744905993,25.5587494649965)) ;
#100683=CARTESIAN_POINT('Ctrl Pts',(38.2925075415833,263.679940643063,25.4920328198283)) ;
#100684=CARTESIAN_POINT('Ctrl Pts',(38.2783336420738,263.677136380134,25.4244712567606)) ;
#100685=CARTESIAN_POINT('Ctrl Pts',(38.2638216154704,263.674265219786,25.3552979710354)) ;
#100686=CARTESIAN_POINT('Ctrl Pts',(38.2530281378403,263.671394059439,25.2852393984215)) ;
#100687=CARTESIAN_POINT('Ctrl Pts',(38.2460487720483,263.668522899092,25.2147288459218)) ;
#100688=CARTESIAN_POINT('Ctrl Pts',(38.2392493059321,263.665725745586,25.1460357688089)) ;
#100689=CARTESIAN_POINT('Ctrl Pts',(38.2360697434519,263.66292859208,25.0769142493217)) ;
#100690=CARTESIAN_POINT('Ctrl Pts',(38.2365467233904,263.660131438574,25.00777484353)) ;
#100691=CARTESIAN_POINT('Ctrl Pts',(38.2370234342225,263.657335863189,24.9386744453718)) ;
#100692=CARTESIAN_POINT('Ctrl Pts',(38.2411525901677,263.654540287804,24.8695566674509)) ;
#100693=CARTESIAN_POINT('Ctrl Pts',(38.24891877186,263.651744712419,24.8008338559926)) ;
#100694=CARTESIAN_POINT('Ctrl Pts',(38.256683176576,263.648949776688,24.7321267689673)) ;
#100695=CARTESIAN_POINT('Ctrl Pts',(38.2680828992034,263.646154840957,24.663814953032)) ;
#100696=CARTESIAN_POINT('Ctrl Pts',(38.2830506609902,263.643359905226,24.5963056594958)) ;
#100697=CARTESIAN_POINT('Ctrl Pts',(38.2987289591487,263.640432290774,24.5255916243843)) ;
#100698=CARTESIAN_POINT('Ctrl Pts',(38.3183224084895,263.637504676322,24.4557587781514)) ;
#100699=CARTESIAN_POINT('Ctrl Pts',(38.3416940811369,263.63457706187,24.3872609126555)) ;
#100700=CARTESIAN_POINT('Ctrl Pts',(38.3640324558406,263.631778881799,24.3217914441699)) ;
#100701=CARTESIAN_POINT('Ctrl Pts',(38.3898217722139,263.628980701728,24.2575418544013)) ;
#100702=CARTESIAN_POINT('Ctrl Pts',(38.4188927833497,263.626182521658,24.1948886568508)) ;
#100703=CARTESIAN_POINT('Ctrl Pts',(38.447982531191,263.623382538118,24.1321950783688)) ;
#100704=CARTESIAN_POINT('Ctrl Pts',(38.4803579551235,263.620582554578,24.0711003701115)) ;
#100705=CARTESIAN_POINT('Ctrl Pts',(38.5158041829826,263.617782571038,24.0119558405473)) ;
#100706=CARTESIAN_POINT('Ctrl Pts',(38.5513048525648,263.614978287014,23.9527204711311)) ;
#100707=CARTESIAN_POINT('Ctrl Pts',(38.5898854610192,263.612174002991,23.8954416574321)) ;
#100708=CARTESIAN_POINT('Ctrl Pts',(38.6312888902081,263.609369718967,23.8404402886788)) ;
#100709=CARTESIAN_POINT('Ctrl Pts',(38.6369051855656,263.608989323245,23.8329794590316)) ;
#100710=CARTESIAN_POINT('Ctrl Pts',(38.6425733641873,263.608608927523,23.8255604821681)) ;
#100711=CARTESIAN_POINT('Ctrl Pts',(38.6482927310412,263.608228531801,23.8181841079402)) ;
#100712=CARTESIAN_POINT('Ctrl Pts',(38.6904563559798,263.605424224442,23.7638048935454)) ;
#100713=CARTESIAN_POINT('Ctrl Pts',(38.7355588715066,263.602619917084,23.7115455412858)) ;
#100714=CARTESIAN_POINT('Ctrl Pts',(38.7833594549891,263.599815609725,23.6617388578696)) ;
#100715=CARTESIAN_POINT('Ctrl Pts',(38.8322994807614,263.596944454931,23.6107449119291)) ;
#100716=CARTESIAN_POINT('Ctrl Pts',(38.8840676143003,263.594073300138,23.5623225303503)) ;
#100717=CARTESIAN_POINT('Ctrl Pts',(38.9383599238844,263.591202145344,23.5167949804171)) ;
#100718=CARTESIAN_POINT('Ctrl Pts',(38.9912537318354,263.588404947888,23.4724401629284)) ;
#100719=CARTESIAN_POINT('Ctrl Pts',(39.0465428414221,263.585607750432,23.4308331693517)) ;
#100720=CARTESIAN_POINT('Ctrl Pts',(39.1039088641049,263.582810552976,23.3922357933253)) ;
#100721=CARTESIAN_POINT('Ctrl Pts',(39.1612425158913,263.580014933942,23.3536601972934)) ;
#100722=CARTESIAN_POINT('Ctrl Pts',(39.2206503513546,263.577219314908,23.318091120167)) ;
#100723=CARTESIAN_POINT('Ctrl Pts',(39.2817831457197,263.574423695874,23.2857483748658)) ;
#100724=CARTESIAN_POINT('Ctrl Pts',(39.3429019443822,263.571628716867,23.253413034092)) ;
#100725=CARTESIAN_POINT('Ctrl Pts',(39.4057444868051,263.56883373786,23.2243027857003)) ;
#100726=CARTESIAN_POINT('Ctrl Pts',(39.4699365096433,263.566038758853,23.1985917433428)) ;
#100727=CARTESIAN_POINT('Ctrl Pts',(39.5371737837546,263.563111186839,23.1716609764619)) ;
#100728=CARTESIAN_POINT('Ctrl Pts',(39.605891241258,263.560183614824,23.1484602140269)) ;
#100729=CARTESIAN_POINT('Ctrl Pts',(39.6756369456841,263.55725604281,23.1291322880882)) ;
#100730=CARTESIAN_POINT('Ctrl Pts',(39.7423010474188,263.554457820895,23.1106583357251)) ;
#100731=CARTESIAN_POINT('Ctrl Pts',(39.8099039370277,263.551659598979,23.0957222547113)) ;
#100732=CARTESIAN_POINT('Ctrl Pts',(39.8780392297342,263.548861377064,23.0843966196071)) ;
#100733=CARTESIAN_POINT('Ctrl Pts',(39.946218423042,263.546061352212,23.0730636872247)) ;
#100734=CARTESIAN_POINT('Ctrl Pts',(40.0149302181711,263.54326132736,23.0653458847454)) ;
#100735=CARTESIAN_POINT('Ctrl Pts',(40.0837633136764,263.540461302508,23.0612638946907)) ;
#100736=CARTESIAN_POINT('Ctrl Pts',(40.1527021026324,263.537656978209,23.0571756367265)) ;
#100737=CARTESIAN_POINT('Ctrl Pts',(40.2217620773208,263.534852653909,23.0567343287276)) ;
#100738=CARTESIAN_POINT('Ctrl Pts',(40.2905332312581,263.53204832961,23.059908611149)) ;
#100739=CARTESIAN_POINT('Ctrl Pts',(40.299855622657,263.531668184633,23.060338906432)) ;
#100740=CARTESIAN_POINT('Ctrl Pts',(40.3091727180629,263.531288039656,23.060835562883)) ;
#100741=CARTESIAN_POINT('Ctrl Pts',(40.3184835082875,263.530907894679,23.0613984297416)) ;
#100742=CARTESIAN_POINT('Ctrl Pts',(40.3871687771503,263.528103582765,23.065550672525)) ;
#100743=CARTESIAN_POINT('Ctrl Pts',(40.4557607972916,263.525299270852,23.073325400445)) ;
#100744=CARTESIAN_POINT('Ctrl Pts',(40.5238489197198,263.522494958938,23.0847114188677)) ;
#100745=CARTESIAN_POINT('Ctrl Pts',(40.593559959848,263.519623804714,23.0963688292773)) ;
#100746=CARTESIAN_POINT('Ctrl Pts',(40.6627422533621,263.51675265049,23.1118119564516)) ;
#100747=CARTESIAN_POINT('Ctrl Pts',(40.7309574422995,263.513881496266,23.1309721099088)) ;
#100748=CARTESIAN_POINT('Ctrl Pts',(40.7974156483534,263.511084292857,23.1496387653313)) ;
#100749=CARTESIAN_POINT('Ctrl Pts',(40.8629554689667,263.508287089447,23.1718331328687)) ;
#100750=CARTESIAN_POINT('Ctrl Pts',(40.927181157058,263.505489886038,23.1974399157849)) ;
#100751=CARTESIAN_POINT('Ctrl Pts',(40.9913706149098,263.502694260555,23.2230322537039)) ;
#100752=CARTESIAN_POINT('Ctrl Pts',(41.0542469594534,263.499898635071,23.2520330067409)) ;
#100753=CARTESIAN_POINT('Ctrl Pts',(41.1154317225032,263.497103009588,23.2842777386029)) ;
#100754=CARTESIAN_POINT('Ctrl Pts',(41.1766024885195,263.49430802365,23.3165150939454)) ;
#100755=CARTESIAN_POINT('Ctrl Pts',(41.2360820107478,263.491513037712,23.3519947267641)) ;
#100756=CARTESIAN_POINT('Ctrl Pts',(41.2935154402097,263.488718051774,23.3905057520064)) ;
#100757=CARTESIAN_POINT('Ctrl Pts',(41.3536732262298,263.48579048559,23.4308435489592)) ;
#100758=CARTESIAN_POINT('Ctrl Pts',(41.4115854696119,263.482862919405,23.4745071977217)) ;
#100759=CARTESIAN_POINT('Ctrl Pts',(41.4668793564282,263.47993535322,23.5212040326503)) ;
#100760=CARTESIAN_POINT('Ctrl Pts',(41.5197304281352,263.477137123266,23.5658378595235)) ;
#100761=CARTESIAN_POINT('Ctrl Pts',(41.5701892879359,263.474338893312,23.6132421229446)) ;
#100762=CARTESIAN_POINT('Ctrl Pts',(41.617966825027,263.471540663358,23.6631221499506)) ;
#100763=CARTESIAN_POINT('Ctrl Pts',(41.6657751521819,263.468740630095,23.7130343219625)) ;
#100764=CARTESIAN_POINT('Ctrl Pts',(41.7108983998769,263.465940596832,23.7654250638381)) ;
#100765=CARTESIAN_POINT('Ctrl Pts',(41.753087537975,263.463140563568,23.8199663784907)) ;
#100766=CARTESIAN_POINT('Ctrl Pts',(41.7953414643923,263.460336230396,23.8745914502492)) ;
#100767=CARTESIAN_POINT('Ctrl Pts',(41.8346520180536,263.457531897224,23.9313732817699)) ;
#100768=CARTESIAN_POINT('Ctrl Pts',(41.8708138762976,263.454727564052,23.9899555968422)) ;
#100769=CARTESIAN_POINT('Ctrl Pts',(41.8757152912741,263.454347461887,23.9978959032975)) ;
#100770=CARTESIAN_POINT('Ctrl Pts',(41.8805589307958,263.453967359722,24.0058692526742)) ;
#100771=CARTESIAN_POINT('Ctrl Pts',(41.8853443503933,263.453587257557,24.0138747268648)) ;
#100772=CARTESIAN_POINT('Ctrl Pts',(41.9216214507285,263.450705795629,24.0745622767291)) ;
#100773=CARTESIAN_POINT('Ctrl Pts',(41.9546748140438,263.447824333702,24.1373083768965)) ;
#100774=CARTESIAN_POINT('Ctrl Pts',(41.9842740327424,263.444942871774,24.2017482441801)) ;
#100775=CARTESIAN_POINT('Ctrl Pts',(42.0138089006307,263.44206767435,24.2660480146013)) ;
#100776=CARTESIAN_POINT('Ctrl Pts',(42.0399043812239,263.439192476926,24.3320338182222)) ;
#100777=CARTESIAN_POINT('Ctrl Pts',(42.0623754778071,263.436317279502,24.3993156573531)) ;
#100778=CARTESIAN_POINT('Ctrl Pts',(42.084817624012,263.433445786306,24.466510814702)) ;
#100779=CARTESIAN_POINT('Ctrl Pts',(42.1036445214476,263.430574293109,24.5349982659407)) ;
#100780=CARTESIAN_POINT('Ctrl Pts',(42.1187190636676,263.427702799912,24.6043678226193)) ;
#100781=CARTESIAN_POINT('Ctrl Pts',(42.1337749073975,263.424834868521,24.6736513331708)) ;
#100782=CARTESIAN_POINT('Ctrl Pts',(42.1450875590401,263.42196693713,24.7438143345802)) ;
#100783=CARTESIAN_POINT('Ctrl Pts',(42.152570042604,263.419099005739,24.8144327443052)) ;
#100784=CARTESIAN_POINT('Ctrl Pts',(42.159863312118,263.41630359745,24.8832653839454)) ;
#100785=CARTESIAN_POINT('Ctrl Pts',(42.1635177960648,263.41350818916,24.9525302509306)) ;
#100786=CARTESIAN_POINT('Ctrl Pts',(42.163499934776,263.41071278087,25.0218264412157)) ;
#100787=CARTESIAN_POINT('',(41.0528501317078,263.,23.252711030329)) ;
#100788=CARTESIAN_POINT('Ctrl Pts',(42.1634999347757,263.410712780838,25.0218264420184)) ;
#100789=CARTESIAN_POINT('Ctrl Pts',(42.1634807839659,263.407715558845,25.096125450968)) ;
#100790=CARTESIAN_POINT('Ctrl Pts',(42.1592401502437,263.404718336852,25.1703150629735)) ;
#100791=CARTESIAN_POINT('Ctrl Pts',(42.1508405655625,263.401721114859,25.2439261335915)) ;
#100792=CARTESIAN_POINT('Ctrl Pts',(42.1424229803534,263.398717469742,25.317694954644)) ;
#100793=CARTESIAN_POINT('Ctrl Pts',(42.1298287214177,263.395713824625,25.3908823956159)) ;
#100794=CARTESIAN_POINT('Ctrl Pts',(42.1131713889199,263.392710179507,25.4630300747387)) ;
#100795=CARTESIAN_POINT('Ctrl Pts',(42.0964543875685,263.389695774921,25.5354361967606)) ;
#100796=CARTESIAN_POINT('Ctrl Pts',(42.0756452976501,263.386681370334,25.6067947481036)) ;
#100797=CARTESIAN_POINT('Ctrl Pts',(42.05090791895,263.383666965747,25.6766615719043)) ;
#100798=CARTESIAN_POINT('Ctrl Pts',(42.0306645464762,263.381200183976,25.7338357840512)) ;
#100799=CARTESIAN_POINT('Ctrl Pts',(42.0077914895878,263.378733402206,25.790011317915)) ;
#100800=CARTESIAN_POINT('Ctrl Pts',(41.9824016122412,263.376266620435,25.8449566362763)) ;
#100801=CARTESIAN_POINT('Ctrl Pts',(41.9535344890115,263.373462002973,25.9074269371122)) ;
#100802=CARTESIAN_POINT('Ctrl Pts',(41.9213266109815,263.370657385511,25.9684916627149)) ;
#100803=CARTESIAN_POINT('Ctrl Pts',(41.8859379059561,263.367852768049,26.0277723430411)) ;
#100804=CARTESIAN_POINT('Ctrl Pts',(41.849710120996,263.364981652018,26.0884585913118)) ;
#100805=CARTESIAN_POINT('Ctrl Pts',(41.8101488762589,263.362110535988,26.1472746069963)) ;
#100806=CARTESIAN_POINT('Ctrl Pts',(41.7674776545232,263.359239419957,26.2038371732794)) ;
#100807=CARTESIAN_POINT('Ctrl Pts',(41.7259004790425,263.35644191639,26.2589495335149)) ;
#100808=CARTESIAN_POINT('Ctrl Pts',(41.6813712050567,263.353644412822,26.311922199575)) ;
#100809=CARTESIAN_POINT('Ctrl Pts',(41.6341412921688,263.350846909255,26.3624284689903)) ;
#100810=CARTESIAN_POINT('Ctrl Pts',(41.5869380671934,263.348050986455,26.4129061991428)) ;
#100811=CARTESIAN_POINT('Ctrl Pts',(41.5370375639455,263.345255063655,26.4609199431382)) ;
#100812=CARTESIAN_POINT('Ctrl Pts',(41.4847307237625,263.342459140856,26.5061769755011)) ;
#100813=CARTESIAN_POINT('Ctrl Pts',(41.4324359106992,263.339663860934,26.5514236017346)) ;
#100814=CARTESIAN_POINT('Ctrl Pts',(41.3777362281772,263.336868581012,26.59391445679)) ;
#100815=CARTESIAN_POINT('Ctrl Pts',(41.3209572868056,263.33407330109,26.6333957174666)) ;
#100816=CARTESIAN_POINT('Ctrl Pts',(41.2614971739138,263.331146024608,26.6747413318834)) ;
#100817=CARTESIAN_POINT('Ctrl Pts',(41.1997570162666,263.328218748127,26.7127857086607)) ;
#100818=CARTESIAN_POINT('Ctrl Pts',(41.1361448941024,263.325291471645,26.747288184293)) ;
#100819=CARTESIAN_POINT('Ctrl Pts',(41.0753309252333,263.322492959431,26.7802729741039)) ;
#100820=CARTESIAN_POINT('Ctrl Pts',(41.0128067100144,263.319694447218,26.8100207603668)) ;
#100821=CARTESIAN_POINT('Ctrl Pts',(40.9489519795987,263.316895935004,26.8363694289166)) ;
#100822=CARTESIAN_POINT('Ctrl Pts',(40.885056200698,263.31409562379,26.8627350354898)) ;
#100823=CARTESIAN_POINT('Ctrl Pts',(40.8198286636425,263.311295312576,26.8856970139188)) ;
#100824=CARTESIAN_POINT('Ctrl Pts',(40.7536655601216,263.308495001361,26.9051427071426)) ;
#100825=CARTESIAN_POINT('Ctrl Pts',(40.6874010513169,263.305690398233,26.9246182039265)) ;
#100826=CARTESIAN_POINT('Ctrl Pts',(40.6201985891142,263.302885795105,26.9405665547925)) ;
#100827=CARTESIAN_POINT('Ctrl Pts',(40.5524648073253,263.300081191977,26.9529261029207)) ;
#100828=CARTESIAN_POINT('Ctrl Pts',(40.54332602458,263.299702789088,26.9545936788657)) ;
#100829=CARTESIAN_POINT('Ctrl Pts',(40.5341775761182,263.2993243862,26.9561960017459)) ;
#100830=CARTESIAN_POINT('Ctrl Pts',(40.5250204651575,263.298945983311,26.9577329925652)) ;
#100831=CARTESIAN_POINT('Ctrl Pts',(40.4571563191861,263.296141606585,26.9691237652409)) ;
#100832=CARTESIAN_POINT('Ctrl Pts',(40.3885690018021,263.293337229859,26.9769634517495)) ;
#100833=CARTESIAN_POINT('Ctrl Pts',(40.319661207915,263.290532853132,26.9811707065517)) ;
#100834=CARTESIAN_POINT('Ctrl Pts',(40.2491127885888,263.28766170701,26.9854781318697)) ;
#100835=CARTESIAN_POINT('Ctrl Pts',(40.1782289285393,263.284790560887,26.9859777612289)) ;
#100836=CARTESIAN_POINT('Ctrl Pts',(40.1074522042496,263.281919414764,26.9826380525251)) ;
#100837=CARTESIAN_POINT('Ctrl Pts',(40.0384964386557,263.279122138103,26.979384268561)) ;
#100838=CARTESIAN_POINT('Ctrl Pts',(39.9696428813651,263.276324861442,26.9724863579311)) ;
#100839=CARTESIAN_POINT('Ctrl Pts',(39.9013030913024,263.273527584781,26.9619677630396)) ;
#100840=CARTESIAN_POINT('Ctrl Pts',(39.8330017813659,263.270731883183,26.9514550908596)) ;
#100841=CARTESIAN_POINT('Ctrl Pts',(39.7652141453778,263.267936181586,26.9373258542111)) ;
#100842=CARTESIAN_POINT('Ctrl Pts',(39.6983459439994,263.265140479989,26.9196552608221)) ;
#100843=CARTESIAN_POINT('Ctrl Pts',(39.6314929752019,263.262345415253,26.9019886927956)) ;
#100844=CARTESIAN_POINT('Ctrl Pts',(39.5655594959524,263.259550350517,26.8807824950459)) ;
#100845=CARTESIAN_POINT('Ctrl Pts',(39.5009386864303,263.256755285781,26.8561624429977)) ;
#100846=CARTESIAN_POINT('Ctrl Pts',(39.4332561415014,263.253827790816,26.8303758923303)) ;
#100847=CARTESIAN_POINT('Ctrl Pts',(39.3670143043893,263.25090029585,26.8008441137367)) ;
#100848=CARTESIAN_POINT('Ctrl Pts',(39.3026421698098,263.247972800884,26.7677685032816)) ;
#100849=CARTESIAN_POINT('Ctrl Pts',(39.2411105635351,263.245174486539,26.7361524095616)) ;
#100850=CARTESIAN_POINT('Ctrl Pts',(39.181287536387,263.242376172193,26.7012989643614)) ;
#100851=CARTESIAN_POINT('Ctrl Pts',(39.1235210375826,263.239577857848,26.6634303561571)) ;
#100852=CARTESIAN_POINT('Ctrl Pts',(39.0657172749725,263.236777738377,26.6255373198069)) ;
#100853=CARTESIAN_POINT('Ctrl Pts',(39.0099730734674,263.233977618905,26.5846255377044)) ;
#100854=CARTESIAN_POINT('Ctrl Pts',(38.9566048140936,263.231177499433,26.5409586760798)) ;
#100855=CARTESIAN_POINT('Ctrl Pts',(38.9031545655358,263.228373078163,26.4972247294426)) ;
#100856=CARTESIAN_POINT('Ctrl Pts',(38.8520878984263,263.225568656893,26.4507275889612)) ;
#100857=CARTESIAN_POINT('Ctrl Pts',(38.8036849584539,263.222764235622,26.4017682979397)) ;
#100858=CARTESIAN_POINT('Ctrl Pts',(38.797132733531,263.222384605811,26.395140760707)) ;
#100859=CARTESIAN_POINT('Ctrl Pts',(38.7906292596009,263.222004976001,26.3884681548245)) ;
#100860=CARTESIAN_POINT('Ctrl Pts',(38.7841751736792,263.22162534619,26.3817512720428)) ;
#100861=CARTESIAN_POINT('Ctrl Pts',(38.7365312003997,263.218822924161,26.3321673359669)) ;
#100862=CARTESIAN_POINT('Ctrl Pts',(38.6914074066215,263.216020502133,26.2799863446704)) ;
#100863=CARTESIAN_POINT('Ctrl Pts',(38.6490979521542,263.213218080105,26.2254943708446)) ;
#100864=CARTESIAN_POINT('Ctrl Pts',(38.6057472495523,263.210346689645,26.1696613334949)) ;
#100865=CARTESIAN_POINT('Ctrl Pts',(38.5653516687552,263.207475299185,26.11140236663)) ;
#100866=CARTESIAN_POINT('Ctrl Pts',(38.5281873948101,263.204603908725,26.0510653911942)) ;
#100867=CARTESIAN_POINT('Ctrl Pts',(38.4920078828847,263.201808603063,25.9923271974779)) ;
#100868=CARTESIAN_POINT('Ctrl Pts',(38.4588908284484,263.199013297401,25.9316202001215)) ;
#100869=CARTESIAN_POINT('Ctrl Pts',(38.4290488774882,263.196217991739,25.8692969774795)) ;
#100870=CARTESIAN_POINT('Ctrl Pts',(38.3992237459258,263.193424261555,25.8070088811964)) ;
#100871=CARTESIAN_POINT('Ctrl Pts',(38.3726702652924,263.190630531372,25.7431068067474)) ;
#100872=CARTESIAN_POINT('Ctrl Pts',(38.3495550741375,263.187836801189,25.6779677575877)) ;
#100873=CARTESIAN_POINT('Ctrl Pts',(38.3264451281523,263.185043704943,25.612843489416)) ;
#100874=CARTESIAN_POINT('Ctrl Pts',(38.3067720850511,263.182250608697,25.5464832639704)) ;
#100875=CARTESIAN_POINT('Ctrl Pts',(38.2906537335265,263.179457512451,25.4792822248378)) ;
#100876=CARTESIAN_POINT('Ctrl Pts',(38.2737488010264,263.176528112169,25.4088017523931)) ;
#100877=CARTESIAN_POINT('Ctrl Pts',(38.2607545537579,263.173598711887,25.337396860385)) ;
#100878=CARTESIAN_POINT('Ctrl Pts',(38.2517467833031,263.170669311605,25.265536750933)) ;
#100879=CARTESIAN_POINT('Ctrl Pts',(38.2431480558051,263.167872935423,25.1969398098517)) ;
#100880=CARTESIAN_POINT('Ctrl Pts',(38.2381815811983,263.16507655924,25.1279286122452)) ;
#100881=CARTESIAN_POINT('Ctrl Pts',(38.2368599469755,263.162280183058,25.0589153194325)) ;
#100882=CARTESIAN_POINT('Ctrl Pts',(38.2355374538086,263.159481989481,24.9898571741492)) ;
#100883=CARTESIAN_POINT('Ctrl Pts',(38.2378644985265,263.156683795904,24.9207974184139)) ;
#100884=CARTESIAN_POINT('Ctrl Pts',(38.2438016143948,263.153885602327,24.8521455045452)) ;
#100885=CARTESIAN_POINT('Ctrl Pts',(38.2497479229573,263.151083076185,24.7833872939384)) ;
#100886=CARTESIAN_POINT('Ctrl Pts',(38.2593153828646,263.148280550043,24.7150386667268)) ;
#100887=CARTESIAN_POINT('Ctrl Pts',(38.2724132323186,263.145478023902,24.6475001955476)) ;
#100888=CARTESIAN_POINT('Ctrl Pts',(38.2742410952635,263.145086918957,24.6380749025441)) ;
#100889=CARTESIAN_POINT('Ctrl Pts',(38.2761376346203,263.144695814012,24.6286653638711)) ;
#100890=CARTESIAN_POINT('Ctrl Pts',(38.2781025269689,263.144304709068,24.6192726434584)) ;
#100891=CARTESIAN_POINT('Ctrl Pts',(38.2922100313937,263.141496659689,24.5518349312221)) ;
#100892=CARTESIAN_POINT('Ctrl Pts',(38.3098966282719,263.138688610311,24.4850193546318)) ;
#100893=CARTESIAN_POINT('Ctrl Pts',(38.3310909267631,263.135880560933,24.4192313750733)) ;
#100894=CARTESIAN_POINT('Ctrl Pts',(38.3527579951909,263.133009873892,24.3519758980682)) ;
#100895=CARTESIAN_POINT('Ctrl Pts',(38.3780911242255,263.130139186851,24.285794934149)) ;
#100896=CARTESIAN_POINT('Ctrl Pts',(38.4069586104773,263.12726849981,24.221111105011)) ;
#100897=CARTESIAN_POINT('Ctrl Pts',(38.4351245577882,263.124467576333,24.1579992251792)) ;
#100898=CARTESIAN_POINT('Ctrl Pts',(38.4666548105774,263.121666652857,24.0963130076055)) ;
#100899=CARTESIAN_POINT('Ctrl Pts',(38.5013772528305,263.118865729381,24.0364279571546)) ;
#100900=CARTESIAN_POINT('Ctrl Pts',(38.5360799229529,263.116066400844,23.9765770072731)) ;
#100901=CARTESIAN_POINT('Ctrl Pts',(38.5739709316143,263.113267072309,23.9185256085515)) ;
#100902=CARTESIAN_POINT('Ctrl Pts',(38.6148320652173,263.110467743773,23.8626250132261)) ;
#100903=CARTESIAN_POINT('Ctrl Pts',(38.65568352523,263.107669077958,23.8067376519794)) ;
#100904=CARTESIAN_POINT('Ctrl Pts',(38.6995034266407,263.104870412144,23.753000474716)) ;
#100905=CARTESIAN_POINT('Ctrl Pts',(38.7460310326053,263.102071746329,23.7017346161992)) ;
#100906=CARTESIAN_POINT('Ctrl Pts',(38.7946418587462,263.099147773464,23.6481733876843)) ;
#100907=CARTESIAN_POINT('Ctrl Pts',(38.8462082137692,263.096223800599,23.5973104412322)) ;
#100908=CARTESIAN_POINT('Ctrl Pts',(38.9003884029964,263.093299827733,23.5494705051135)) ;
#100909=CARTESIAN_POINT('Ctrl Pts',(38.9523049486173,263.090498018201,23.5036293173762)) ;
#100910=CARTESIAN_POINT('Ctrl Pts',(39.0066208255902,263.087696208668,23.4605638308037)) ;
#100911=CARTESIAN_POINT('Ctrl Pts',(39.0630019956775,263.084894399136,23.4205181108754)) ;
#100912=CARTESIAN_POINT('Ctrl Pts',(39.1194186886288,263.082090824328,23.3804471602068)) ;
#100913=CARTESIAN_POINT('Ctrl Pts',(39.1779028545884,263.079287249519,23.3434000232094)) ;
#100914=CARTESIAN_POINT('Ctrl Pts',(39.2380932403682,263.076483674711,23.3095763101905)) ;
#100915=CARTESIAN_POINT('Ctrl Pts',(39.2983742689995,263.0736758779,23.2757016608343)) ;
#100916=CARTESIAN_POINT('Ctrl Pts',(39.3603662077959,263.070868081088,23.2450603323664)) ;
#100917=CARTESIAN_POINT('Ctrl Pts',(39.4236860971042,263.068060284276,23.2178046174927)) ;
#100918=CARTESIAN_POINT('Ctrl Pts',(39.4317761466145,263.067701546833,23.2143222980323)) ;
#100919=CARTESIAN_POINT('Ctrl Pts',(39.4398878519879,263.067342809389,23.2108951783485)) ;
#100920=CARTESIAN_POINT('Ctrl Pts',(39.4480203969485,263.066984071946,23.2075235173978)) ;
#100921=CARTESIAN_POINT('Ctrl Pts',(39.5112921790507,263.064193068948,23.1812917537828)) ;
#100922=CARTESIAN_POINT('Ctrl Pts',(39.576070983772,263.06140206595,23.1583198387983)) ;
#100923=CARTESIAN_POINT('Ctrl Pts',(39.6419825877609,263.058611062953,23.1387824773699)) ;
#100924=CARTESIAN_POINT('Ctrl Pts',(39.7071246471384,263.055852646043,23.1194732225312)) ;
#100925=CARTESIAN_POINT('Ctrl Pts',(39.7733727088633,263.053094229133,23.1035189237572)) ;
#100926=CARTESIAN_POINT('Ctrl Pts',(39.8403441402275,263.050335812223,23.0910405937484)) ;
#100927=CARTESIAN_POINT('Ctrl Pts',(39.9072570590145,263.047579805327,23.078573165989)) ;
#100928=CARTESIAN_POINT('Ctrl Pts',(39.9748916016868,263.044823798431,23.0695757791274)) ;
#100929=CARTESIAN_POINT('Ctrl Pts',(40.0428519602401,263.042067791535,23.0641190908521)) ;
#100930=CARTESIAN_POINT('Ctrl Pts',(40.1107774956255,263.039313196828,23.0586651986064)) ;
#100931=CARTESIAN_POINT('Ctrl Pts',(40.1790280144218,263.036558602122,23.0567484464848)) ;
#100932=CARTESIAN_POINT('Ctrl Pts',(40.247201510416,263.033804007415,23.0583877753305)) ;
#100933=CARTESIAN_POINT('Ctrl Pts',(40.3169194910234,263.030987006797,23.0600642435093)) ;
#100934=CARTESIAN_POINT('Ctrl Pts',(40.3865563712997,263.028170006179,23.0654599469317)) ;
#100935=CARTESIAN_POINT('Ctrl Pts',(40.4556830337894,263.025353005561,23.0745387851324)) ;
#100936=CARTESIAN_POINT('Ctrl Pts',(40.5233155646348,263.022596892734,23.0834213896519)) ;
#100937=CARTESIAN_POINT('Ctrl Pts',(40.5904592123026,263.019840779907,23.0958293517773)) ;
#100938=CARTESIAN_POINT('Ctrl Pts',(40.6567205532952,263.01708466708,23.1116767678634)) ;
#100939=CARTESIAN_POINT('Ctrl Pts',(40.7251776534542,263.014237222567,23.1280493334351)) ;
#100940=CARTESIAN_POINT('Ctrl Pts',(40.7926923736418,263.011389778053,23.1480931961573)) ;
#100941=CARTESIAN_POINT('Ctrl Pts',(40.8588485940152,263.00854233354,23.1716580013565)) ;
#100942=CARTESIAN_POINT('Ctrl Pts',(40.9250048143885,263.005694889027,23.1952228065557)) ;
#100943=CARTESIAN_POINT('Ctrl Pts',(40.9898020147256,263.002847444513,23.2223082757636)) ;
#100944=CARTESIAN_POINT('Ctrl Pts',(41.0528501317078,263.,23.252711030329)) ;
#100945=CARTESIAN_POINT('Ctrl Pts',(41.0528501317078,263.,23.252711030329)) ;
#100946=CARTESIAN_POINT('Ctrl Pts',(41.0637961405579,263.,23.2581157538237)) ;
#100947=CARTESIAN_POINT('Ctrl Pts',(41.074742149408,263.,23.2635204773184)) ;
#100948=CARTESIAN_POINT('Ctrl Pts',(41.0856881582581,263.,23.2689252008131)) ;
#100949=CARTESIAN_POINT('',(42.1635,255.,25.0213203435596)) ;
#100950=CARTESIAN_POINT('Origin',(40.2,255.,25.0213203435596)) ;
#100951=CARTESIAN_POINT('Origin',(40.2,265.924309379709,25.0213203435596)) ;
#100952=CARTESIAN_POINT('',(39.2427274574787,263.,26.3991716932468)) ;
#100953=CARTESIAN_POINT('Ctrl Pts',(39.2427274574787,263.,26.3991716932468)) ;
#100954=CARTESIAN_POINT('Ctrl Pts',(39.2911023455816,263.003084054089,26.4327805089866)) ;
#100955=CARTESIAN_POINT('Ctrl Pts',(39.3412181789107,263.006211645544,26.4638215959221)) ;
#100956=CARTESIAN_POINT('Ctrl Pts',(39.4699166383487,263.01394653045,26.5344454303808)) ;
#100957=CARTESIAN_POINT('Ctrl Pts',(39.5501746528686,263.018506385508,26.5706101629425)) ;
#100958=CARTESIAN_POINT('Ctrl Pts',(39.6661076125514,263.024630231193,26.6122473389269)) ;
#100959=CARTESIAN_POINT('Ctrl Pts',(39.6996808889019,263.026353491027,26.6231227004272)) ;
#100960=CARTESIAN_POINT('Ctrl Pts',(39.7610537645275,263.029415612689,26.6408849987459)) ;
#100961=CARTESIAN_POINT('Ctrl Pts',(39.7887336180132,263.030765067584,26.6481342687505)) ;
#100962=CARTESIAN_POINT('Ctrl Pts',(39.8517601410882,263.033771737349,26.6629291376098)) ;
#100963=CARTESIAN_POINT('Ctrl Pts',(39.8871926527789,263.03541569227,26.6700477922631)) ;
#100964=CARTESIAN_POINT('Ctrl Pts',(40.025705529455,263.041693627517,26.6932494861919)) ;
#100965=CARTESIAN_POINT('Ctrl Pts',(40.1299691561863,263.046085821433,26.700850832178)) ;
#100966=CARTESIAN_POINT('Ctrl Pts',(40.3167787214546,263.053989498904,26.6970349195049)) ;
#100967=CARTESIAN_POINT('Ctrl Pts',(40.3990509823152,263.057489072505,26.6892631852092)) ;
#100968=CARTESIAN_POINT('Ctrl Pts',(40.5025796865608,263.062241845599,26.6717130852496)) ;
#100969=CARTESIAN_POINT('Ctrl Pts',(40.5246704101568,263.063276871209,26.6675097953225)) ;
#100970=CARTESIAN_POINT('Ctrl Pts',(40.5627942014101,263.065109280979,26.6594586303915)) ;
#100971=CARTESIAN_POINT('Ctrl Pts',(40.5788664978773,263.065896700378,26.6558162329867)) ;
#100972=CARTESIAN_POINT('Ctrl Pts',(40.6180174490815,263.067851580907,26.646335132263)) ;
#100973=CARTESIAN_POINT('Ctrl Pts',(40.6410290389475,263.069031077354,26.6402412613374)) ;
#100974=CARTESIAN_POINT('Ctrl Pts',(40.7671234650463,263.075634532828,26.6039613959264)) ;
#100975=CARTESIAN_POINT('Ctrl Pts',(40.8672505236624,263.08138241966,26.5644202025094)) ;
#100976=CARTESIAN_POINT('Ctrl Pts',(41.0389529161193,263.091519303937,26.476756175076)) ;
#100977=CARTESIAN_POINT('Ctrl Pts',(41.1119297697296,263.0959336199,26.4321789667875)) ;
#100978=CARTESIAN_POINT('Ctrl Pts',(41.2090558997039,263.101870477116,26.3621523481488)) ;
#100979=CARTESIAN_POINT('Ctrl Pts',(41.2362885731461,263.103543880883,26.3412182438542)) ;
#100980=CARTESIAN_POINT('Ctrl Pts',(41.2849477404721,263.106552212936,26.3013782803977)) ;
#100981=CARTESIAN_POINT('Ctrl Pts',(41.3065702733717,263.107896150544,26.2827331486183)) ;
#100982=CARTESIAN_POINT('Ctrl Pts',(41.3545780272055,263.110901574535,26.2391510886397)) ;
#100983=CARTESIAN_POINT('Ctrl Pts',(41.3806510884628,263.112549377426,26.2138912467673)) ;
#100984=CARTESIAN_POINT('Ctrl Pts',(41.4751073086673,263.118608432302,26.1162445044194)) ;
#100985=CARTESIAN_POINT('Ctrl Pts',(41.5378247274081,263.122803876602,26.0386619543441)) ;
#100986=CARTESIAN_POINT('Ctrl Pts',(41.6276347117263,263.129600955505,25.9047818671928)) ;
#100987=CARTESIAN_POINT('Ctrl Pts',(41.6591275250957,263.132199923992,25.8517367826009)) ;
#100988=CARTESIAN_POINT('Ctrl Pts',(41.7002796632013,263.13608235282,25.7728218824172)) ;
#100989=CARTESIAN_POINT('Ctrl Pts',(41.7123346684026,263.137293244777,25.7482573250673)) ;
#100990=CARTESIAN_POINT('Ctrl Pts',(41.7331888116543,263.13954664214,25.7029964442953)) ;
#100991=CARTESIAN_POINT('Ctrl Pts',(41.7421828782459,263.140580413658,25.6823968336961)) ;
#100992=CARTESIAN_POINT('Ctrl Pts',(41.7569854939115,263.142403288016,25.6465461595278)) ;
#100993=CARTESIAN_POINT('Ctrl Pts',(41.7629900404973,263.143182096106,25.6313803762269)) ;
#100994=CARTESIAN_POINT('Ctrl Pts',(41.7769827331857,263.145096227955,25.5944754675309)) ;
#100995=CARTESIAN_POINT('Ctrl Pts',(41.7847431952058,263.146242664951,25.5726553129982)) ;
#100996=CARTESIAN_POINT('Ctrl Pts',(41.8214679770377,263.152094654795,25.4622060578001)) ;
#100997=CARTESIAN_POINT('Ctrl Pts',(41.843458699302,263.157051484054,25.371435403534)) ;
#100998=CARTESIAN_POINT('Ctrl Pts',(41.8730849494486,263.167223396867,25.1810649885886)) ;
#100999=CARTESIAN_POINT('Ctrl Pts',(41.8796120584156,263.172409089272,25.0816425807865)) ;
#101000=CARTESIAN_POINT('Ctrl Pts',(41.8764894512499,263.179060704958,24.9476942236183)) ;
#101001=CARTESIAN_POINT('Ctrl Pts',(41.87461879154,263.180745460967,24.9132009903328)) ;
#101002=CARTESIAN_POINT('Ctrl Pts',(41.8692833714942,263.183752319547,24.8506245214068)) ;
#101003=CARTESIAN_POINT('Ctrl Pts',(41.8661706103987,263.185084292789,24.8225248544848)) ;
#101004=CARTESIAN_POINT('Ctrl Pts',(41.8574973326201,263.188060815679,24.7589545102575)) ;
#101005=CARTESIAN_POINT('Ctrl Pts',(41.8515054048496,263.18969189326,24.7235564441324)) ;
#101006=CARTESIAN_POINT('Ctrl Pts',(41.8288396042035,263.194789620036,24.6116119757236)) ;
#101007=CARTESIAN_POINT('Ctrl Pts',(41.8079399838252,263.198135712618,24.5360271352042)) ;
#101008=CARTESIAN_POINT('Ctrl Pts',(41.7478250208186,263.205749223442,24.3659601537163)) ;
#101009=CARTESIAN_POINT('Ctrl Pts',(41.7051096405367,263.209969965747,24.2730547361341)) ;
#101010=CARTESIAN_POINT('Ctrl Pts',(41.6404218902882,263.215739775026,24.1606254410539)) ;
#101011=CARTESIAN_POINT('Ctrl Pts',(41.6260296485181,263.216994073744,24.1369843001121)) ;
#101012=CARTESIAN_POINT('Ctrl Pts',(41.6020403556091,263.219056457892,24.0996881501309)) ;
#101013=CARTESIAN_POINT('Ctrl Pts',(41.5928123968713,263.219843806571,24.0858008718972)) ;
#101014=CARTESIAN_POINT('Ctrl Pts',(41.5722938643976,263.221585631042,24.0558989607961)) ;
#101015=CARTESIAN_POINT('Ctrl Pts',(41.5609272545832,263.222544244534,24.039940782142)) ;
#101016=CARTESIAN_POINT('Ctrl Pts',(41.5245861708713,263.225580659118,23.9907654115108)) ;
#101017=CARTESIAN_POINT('Ctrl Pts',(41.4986562029933,263.22770690375,23.9582758156866)) ;
#101018=CARTESIAN_POINT('Ctrl Pts',(41.4109059869568,263.234694050313,23.8563343013838)) ;
#101019=CARTESIAN_POINT('Ctrl Pts',(41.3445135837078,263.239662808617,23.7910460352389)) ;
#101020=CARTESIAN_POINT('Ctrl Pts',(41.2341691711625,263.247159010316,23.6992394226413)) ;
#101021=CARTESIAN_POINT('Ctrl Pts',(41.1938387993125,263.24976543816,23.6686604539096)) ;
#101022=CARTESIAN_POINT('Ctrl Pts',(41.1182555322,263.254391408475,23.6165605199913)) ;
#101023=CARTESIAN_POINT('Ctrl Pts',(41.0834731061389,263.256428855633,23.5944289685198)) ;
#101024=CARTESIAN_POINT('Ctrl Pts',(41.0230259574888,263.259817367044,23.5590259489106)) ;
#101025=CARTESIAN_POINT('Ctrl Pts',(40.9977704581187,263.261190359206,23.5450957540483)) ;
#101026=CARTESIAN_POINT('Ctrl Pts',(40.9439089115288,263.264033444163,23.5171734933855)) ;
#101027=CARTESIAN_POINT('Ctrl Pts',(40.9152382740148,263.265498213573,23.5033306941647)) ;
#101028=CARTESIAN_POINT('Ctrl Pts',(40.8276193800529,263.269843530878,23.4640603732382)) ;
#101029=CARTESIAN_POINT('Ctrl Pts',(40.7675880952944,263.272644121892,23.4411908274066)) ;
#101030=CARTESIAN_POINT('Ctrl Pts',(40.5980758009466,263.280250569522,23.3875245171677)) ;
#101031=CARTESIAN_POINT('Ctrl Pts',(40.4865646037941,263.284906580776,23.3643256552867)) ;
#101032=CARTESIAN_POINT('Ctrl Pts',(40.3472783566533,263.291026599974,23.3498380828204)) ;
#101033=CARTESIAN_POINT('Ctrl Pts',(40.320925317618,263.292198756319,23.3477251621585)) ;
#101034=CARTESIAN_POINT('Ctrl Pts',(40.2726515134719,263.294388350675,23.3450008024137)) ;
#101035=CARTESIAN_POINT('Ctrl Pts',(40.2507474472316,263.295397806973,23.3441948070596)) ;
#101036=CARTESIAN_POINT('Ctrl Pts',(40.2125000072133,263.297197425772,23.3435373669686)) ;
#101037=CARTESIAN_POINT('Ctrl Pts',(40.1961637934343,263.297978396315,23.3434952037403)) ;
#101038=CARTESIAN_POINT('Ctrl Pts',(40.1560105545898,263.299927803157,23.3439779794298)) ;
#101039=CARTESIAN_POINT('Ctrl Pts',(40.132201616325,263.301108610646,23.3447715799927)) ;
#101040=CARTESIAN_POINT('Ctrl Pts',(40.0428126016676,263.30561579772,23.3496582322217)) ;
#101041=CARTESIAN_POINT('Ctrl Pts',(39.9774771865611,263.309057949274,23.3570953752569)) ;
#101042=CARTESIAN_POINT('Ctrl Pts',(39.8300932341571,263.316947114412,23.3827073434764)) ;
#101043=CARTESIAN_POINT('Ctrl Pts',(39.7486255132985,263.321393499707,23.4032517507411)) ;
#101044=CARTESIAN_POINT('Ctrl Pts',(39.6167153908434,263.328545406163,23.4472599661822)) ;
#101045=CARTESIAN_POINT('Ctrl Pts',(39.5652860976606,263.3313230774,23.4672849376038)) ;
#101046=CARTESIAN_POINT('Ctrl Pts',(39.4869005243371,263.335527213952,23.5023479041454)) ;
#101047=CARTESIAN_POINT('Ctrl Pts',(39.4592163982495,263.337006406119,23.5156550640532)) ;
#101048=CARTESIAN_POINT('Ctrl Pts',(39.4319120248721,263.338461000729,23.5297151930711)) ;
#101049=CARTESIAN_POINT('',(41.1743400212928,263.,26.3871558334365)) ;
#101050=CARTESIAN_POINT('Origin',(40.2,263.,25.0213203435596)) ;
#101051=CARTESIAN_POINT('',(41.8777498381111,263.075690620251,25.020583310179)) ;
#101052=CARTESIAN_POINT('Ctrl Pts',(41.8777498381111,263.075690620251,25.020583310179)) ;
#101053=CARTESIAN_POINT('Ctrl Pts',(41.8777771592572,263.07272122919,25.0827759458533)) ;
#101054=CARTESIAN_POINT('Ctrl Pts',(41.8743420727466,263.069751838128,25.1450776443993)) ;
#101055=CARTESIAN_POINT('Ctrl Pts',(41.8674345209409,263.066782447066,25.2070814290289)) ;
#101056=CARTESIAN_POINT('Ctrl Pts',(41.860540872367,263.063819032671,25.2689604150301)) ;
#101057=CARTESIAN_POINT('Ctrl Pts',(41.8501887092101,263.060855618275,25.3305422015561)) ;
#101058=CARTESIAN_POINT('Ctrl Pts',(41.8364199278902,263.05789220388,25.3914215217578)) ;
#101059=CARTESIAN_POINT('Ctrl Pts',(41.8226673239878,263.054932271303,25.4522293127406)) ;
#101060=CARTESIAN_POINT('Ctrl Pts',(41.8055061776375,263.051972338726,25.5123358062267)) ;
#101061=CARTESIAN_POINT('Ctrl Pts',(41.7850297859598,263.049012406148,25.5713436522658)) ;
#101062=CARTESIAN_POINT('Ctrl Pts',(41.7645710407854,263.046055024434,25.6303006454906)) ;
#101063=CARTESIAN_POINT('Ctrl Pts',(41.740802882733,263.043097642719,25.688160415573)) ;
#101064=CARTESIAN_POINT('Ctrl Pts',(41.7138685664242,263.040140261004,25.7445402451752)) ;
#101065=CARTESIAN_POINT('Ctrl Pts',(41.6869490350041,263.037184502667,25.800889126544)) ;
#101066=CARTESIAN_POINT('Ctrl Pts',(41.6568670075066,263.034228744329,25.8557592455103)) ;
#101067=CARTESIAN_POINT('Ctrl Pts',(41.6238133602854,263.031272985992,25.9087889782576)) ;
#101068=CARTESIAN_POINT('Ctrl Pts',(41.5907565441787,263.028316944283,25.9618237950174)) ;
#101069=CARTESIAN_POINT('Ctrl Pts',(41.5547277859931,263.025360902574,26.0130174561376)) ;
#101070=CARTESIAN_POINT('Ctrl Pts',(41.5159626404356,263.022404860865,26.0620351899405)) ;
#101071=CARTESIAN_POINT('Ctrl Pts',(41.477196741694,263.019448761722,26.1110538761295)) ;
#101072=CARTESIAN_POINT('Ctrl Pts',(41.4356946569183,263.016492662579,26.1578961760627)) ;
#101073=CARTESIAN_POINT('Ctrl Pts',(41.3917324065674,263.013536563436,26.2022601953883)) ;
#101074=CARTESIAN_POINT('Ctrl Pts',(41.3477333703716,263.010577990748,26.2466613367428)) ;
#101075=CARTESIAN_POINT('Ctrl Pts',(41.3012704057273,263.00761941806,26.2885797186237)) ;
#101076=CARTESIAN_POINT('Ctrl Pts',(41.2526557659135,263.004660845372,26.3277509391096)) ;
#101077=CARTESIAN_POINT('Ctrl Pts',(41.2271270912358,263.003107230248,26.3483206553173)) ;
#101078=CARTESIAN_POINT('Ctrl Pts',(41.2010056420111,263.001553615124,26.3681334975468)) ;
#101079=CARTESIAN_POINT('Ctrl Pts',(41.1743400212928,263.,26.3871558334365)) ;
#101080=CARTESIAN_POINT('Ctrl Pts',(39.4319120248721,263.238554795302,23.5297151930711)) ;
#101081=CARTESIAN_POINT('Ctrl Pts',(39.4729859837156,263.236357167323,23.5085645461534)) ;
#101082=CARTESIAN_POINT('Ctrl Pts',(39.5148870253905,263.234159539345,23.4891359763675)) ;
#101083=CARTESIAN_POINT('Ctrl Pts',(39.5574566951772,263.231961911366,23.4714870738407)) ;
#101084=CARTESIAN_POINT('Ctrl Pts',(39.6139302242998,263.229046506848,23.4480737888466)) ;
#101085=CARTESIAN_POINT('Ctrl Pts',(39.6717913139331,263.226131102329,23.4277071800005)) ;
#101086=CARTESIAN_POINT('Ctrl Pts',(39.7306799504516,263.223215697811,23.4105491762016)) ;
#101087=CARTESIAN_POINT('Ctrl Pts',(39.7894735976778,263.220304995935,23.3934188488227)) ;
#101088=CARTESIAN_POINT('Ctrl Pts',(39.8492910166438,263.21739429406,23.379486990035)) ;
#101089=CARTESIAN_POINT('Ctrl Pts',(39.9097534462909,263.214483592184,23.3688670157588)) ;
#101090=CARTESIAN_POINT('Ctrl Pts',(39.9701615273374,263.211575506686,23.3582565875882)) ;
#101091=CARTESIAN_POINT('Ctrl Pts',(40.0312129718539,263.208667421188,23.3509522293592)) ;
#101092=CARTESIAN_POINT('Ctrl Pts',(40.0925167041359,263.205759335691,23.347016785775)) ;
#101093=CARTESIAN_POINT('Ctrl Pts',(40.1537876337663,263.202852806263,23.3430834479841)) ;
#101094=CARTESIAN_POINT('Ctrl Pts',(40.215310077744,263.199946276836,23.3425154816823)) ;
#101095=CARTESIAN_POINT('Ctrl Pts',(40.2766877039282,263.197039747409,23.3453239060436)) ;
#101096=CARTESIAN_POINT('Ctrl Pts',(40.3380548153899,263.194133715904,23.3481318492882)) ;
#101097=CARTESIAN_POINT('Ctrl Pts',(40.3992766515522,263.1912276844,23.3543150106123)) ;
#101098=CARTESIAN_POINT('Ctrl Pts',(40.4599587899172,263.188321652896,23.3638323375563)) ;
#101099=CARTESIAN_POINT('Ctrl Pts',(40.5206952141623,263.185413021674,23.3733581786444)) ;
#101100=CARTESIAN_POINT('Ctrl Pts',(40.5808904733218,263.182504390451,23.3862240666862)) ;
#101101=CARTESIAN_POINT('Ctrl Pts',(40.6401583757575,263.179595759228,23.4023374323618)) ;
#101102=CARTESIAN_POINT('Ctrl Pts',(40.6994516451042,263.176685883099,23.4184576946255)) ;
#101103=CARTESIAN_POINT('Ctrl Pts',(40.7578162835293,263.17377600697,23.4378280462673)) ;
#101104=CARTESIAN_POINT('Ctrl Pts',(40.8148822755349,263.170866130841,23.4603062982246)) ;
#101105=CARTESIAN_POINT('Ctrl Pts',(40.8720526552897,263.167950931833,23.4828256684391)) ;
#101106=CARTESIAN_POINT('Ctrl Pts',(40.9279191788123,263.165035732824,23.5084640873553)) ;
#101107=CARTESIAN_POINT('Ctrl Pts',(40.9821335654524,263.162120533815,23.5370319119222)) ;
#101108=CARTESIAN_POINT('Ctrl Pts',(41.0284978638453,263.159627447291,23.5614631971352)) ;
#101109=CARTESIAN_POINT('Ctrl Pts',(41.0736540897011,263.157134360768,23.5880360870147)) ;
#101110=CARTESIAN_POINT('Ctrl Pts',(41.1174017602243,263.154641274244,23.6166071796584)) ;
#101111=CARTESIAN_POINT('Ctrl Pts',(41.1683248599349,263.151739275301,23.649864461295)) ;
#101112=CARTESIAN_POINT('Ctrl Pts',(41.2175404960184,263.148837276357,23.6859619109233)) ;
#101113=CARTESIAN_POINT('Ctrl Pts',(41.2647134168509,263.145935277414,23.7246976526901)) ;
#101114=CARTESIAN_POINT('Ctrl Pts',(41.3118076620972,263.143038118461,23.7633687905032)) ;
#101115=CARTESIAN_POINT('Ctrl Pts',(41.356865561525,263.140140959508,23.80466916243)) ;
#101116=CARTESIAN_POINT('Ctrl Pts',(41.3995810245911,263.137243800554,23.848353835964)) ;
#101117=CARTESIAN_POINT('Ctrl Pts',(41.4422568256992,263.134349331657,23.8919979476134)) ;
#101118=CARTESIAN_POINT('Ctrl Pts',(41.4825941434519,263.13145486276,23.9380216083587)) ;
#101119=CARTESIAN_POINT('Ctrl Pts',(41.5203214559646,263.128560393863,23.9861409796716)) ;
#101120=CARTESIAN_POINT('Ctrl Pts',(41.5580278495891,263.12566752988,24.0342336699495)) ;
#101121=CARTESIAN_POINT('Ctrl Pts',(41.5931267911853,263.122774665896,24.0844193636267)) ;
#101122=CARTESIAN_POINT('Ctrl Pts',(41.6253864283048,263.119881801913,24.1363804628307)) ;
#101123=CARTESIAN_POINT('Ctrl Pts',(41.6576402441328,263.11698945995,24.18833218559)) ;
#101124=CARTESIAN_POINT('Ctrl Pts',(41.6870555025148,263.114097117987,24.2420582416089)) ;
#101125=CARTESIAN_POINT('Ctrl Pts',(41.713444335914,263.111204776025,24.2972130969519)) ;
#101126=CARTESIAN_POINT('Ctrl Pts',(41.7398575598809,263.108309760739,24.3524189306087)) ;
#101127=CARTESIAN_POINT('Ctrl Pts',(41.7632385472967,263.105414745454,24.4090557383128)) ;
#101128=CARTESIAN_POINT('Ctrl Pts',(41.7834465659634,263.102519730169,24.466755617636)) ;
#101129=CARTESIAN_POINT('Ctrl Pts',(41.8036634105825,263.099623450472,24.5244806976677)) ;
#101130=CARTESIAN_POINT('Ctrl Pts',(41.8207043811825,263.096727170774,24.5832692807788)) ;
#101131=CARTESIAN_POINT('Ctrl Pts',(41.8344788449778,263.093830891077,24.6427388228538)) ;
#101132=CARTESIAN_POINT('Ctrl Pts',(41.8482796054899,263.090929082115,24.7023218977474)) ;
#101133=CARTESIAN_POINT('Ctrl Pts',(41.8588013103894,263.088027273154,24.7625880219625)) ;
#101134=CARTESIAN_POINT('Ctrl Pts',(41.8660047802855,263.085125464192,24.8231458382216)) ;
#101135=CARTESIAN_POINT('Ctrl Pts',(41.8724630318549,263.082523855169,24.8774387855847)) ;
#101136=CARTESIAN_POINT('Ctrl Pts',(41.8762548028084,263.079922246146,24.9319658532433)) ;
#101137=CARTESIAN_POINT('Ctrl Pts',(41.8773874970113,263.077320637123,24.9864456052773)) ;
#101138=CARTESIAN_POINT('Ctrl Pts',(41.877624057104,263.076777298179,24.9978235527949)) ;
#101139=CARTESIAN_POINT('Ctrl Pts',(41.8777448388839,263.076233959235,25.0092033057449)) ;
#101140=CARTESIAN_POINT('Ctrl Pts',(41.8777498381107,263.075690620291,25.0205833093468)) ;
#101141=CARTESIAN_POINT('Origin',(40.2,263.,25.0213203435596)) ;
#101142=CARTESIAN_POINT('Ctrl Pts',(41.0856881582581,263.,23.2689252008131)) ;
#101143=CARTESIAN_POINT('Ctrl Pts',(41.136560203023,263.,23.2988237487254)) ;
#101144=CARTESIAN_POINT('Ctrl Pts',(41.1859148580529,263.,23.331059625684)) ;
#101145=CARTESIAN_POINT('Ctrl Pts',(41.2335581419714,263.,23.3656315345143)) ;
#101146=CARTESIAN_POINT('Ctrl Pts',(41.2443647676521,263.,23.3734732626042)) ;
#101147=CARTESIAN_POINT('Ctrl Pts',(41.2550832802686,263.,23.3814352538179)) ;
#101148=CARTESIAN_POINT('Ctrl Pts',(41.2657112952103,263.,23.3895176261393)) ;
#101149=CARTESIAN_POINT('Ctrl Pts',(41.3262097912653,263.,23.4355254058313)) ;
#101150=CARTESIAN_POINT('Ctrl Pts',(41.3837800806245,263.,23.4854310739318)) ;
#101151=CARTESIAN_POINT('Ctrl Pts',(41.4382345422844,263.,23.5388477209115)) ;
#101152=CARTESIAN_POINT('Ctrl Pts',(41.4520628554996,263.,23.5524124886611)) ;
#101153=CARTESIAN_POINT('Ctrl Pts',(41.4656930103321,263.,23.5662072310807)) ;
#101154=CARTESIAN_POINT('Ctrl Pts',(41.4791016494721,263.,23.5802046256661)) ;
#101155=CARTESIAN_POINT('Ctrl Pts',(41.5290702340151,263.,23.6323672640532)) ;
#101156=CARTESIAN_POINT('Ctrl Pts',(41.576018175633,263.,23.6873903203988)) ;
#101157=CARTESIAN_POINT('Ctrl Pts',(41.61980527048,263.,23.7449249724425)) ;
#101158=CARTESIAN_POINT('Ctrl Pts',(41.6533521475531,263.,23.7890043503116)) ;
#101159=CARTESIAN_POINT('Ctrl Pts',(41.68504294083,263.,23.8345588425587)) ;
#101160=CARTESIAN_POINT('Ctrl Pts',(41.7147961550209,263.,23.8814408944727)) ;
#101161=CARTESIAN_POINT('Ctrl Pts',(41.7260447826157,263.,23.8991653238226)) ;
#101162=CARTESIAN_POINT('Ctrl Pts',(41.7370162940054,263.,23.9170795619092)) ;
#101163=CARTESIAN_POINT('Ctrl Pts',(41.7477056363485,263.,23.9351757974312)) ;
#101164=CARTESIAN_POINT('Ctrl Pts',(41.7567703799348,263.,23.9505217120459)) ;
#101165=CARTESIAN_POINT('Ctrl Pts',(41.7656346827696,263.,23.9660032706815)) ;
#101166=CARTESIAN_POINT('Ctrl Pts',(41.7742803042553,263.,23.9815879252681)) ;
#101167=CARTESIAN_POINT('Ctrl Pts',(41.8089017809343,263.,24.0439968285742)) ;
#101168=CARTESIAN_POINT('Ctrl Pts',(41.8400645548394,263.,24.1081277587535)) ;
#101169=CARTESIAN_POINT('Ctrl Pts',(41.8676322251476,263.,24.173652136793)) ;
#101170=CARTESIAN_POINT('Ctrl Pts',(41.8948232811182,263.,24.2382813568462)) ;
#101171=CARTESIAN_POINT('Ctrl Pts',(41.9185170247662,263.,24.3042672193153)) ;
#101172=CARTESIAN_POINT('Ctrl Pts',(41.9385345807979,263.,24.3713076356331)) ;
#101173=CARTESIAN_POINT('Ctrl Pts',(41.9533071976636,263.,24.4207823259104)) ;
#101174=CARTESIAN_POINT('Ctrl Pts',(41.9660767335746,263.,24.4708316800822)) ;
#101175=CARTESIAN_POINT('Ctrl Pts',(41.9767529969391,263.,24.5213342818128)) ;
#101176=CARTESIAN_POINT('Ctrl Pts',(41.982807227349,263.,24.5499729896388)) ;
#101177=CARTESIAN_POINT('Ctrl Pts',(41.9881880273261,263.,24.5787574266971)) ;
#101178=CARTESIAN_POINT('Ctrl Pts',(41.9928765697548,263.,24.6076650255236)) ;
#101179=CARTESIAN_POINT('Ctrl Pts',(41.9948224733389,263.,24.6196626561349)) ;
#101180=CARTESIAN_POINT('Ctrl Pts',(41.9966494227026,263.,24.631683708088)) ;
#101181=CARTESIAN_POINT('Ctrl Pts',(41.9983549861683,263.,24.6437194565562)) ;
#101182=CARTESIAN_POINT('Ctrl Pts',(42.0079094303121,263.,24.7111428557921)) ;
#101183=CARTESIAN_POINT('Ctrl Pts',(42.013629467554,263.,24.778810574148)) ;
#101184=CARTESIAN_POINT('Ctrl Pts',(42.0153609924019,263.,24.8464405106901)) ;
#101185=CARTESIAN_POINT('Ctrl Pts',(42.0165329099533,263.,24.89221329283)) ;
#101186=CARTESIAN_POINT('Ctrl Pts',(42.0158767839533,263.,24.9379689419043)) ;
#101187=CARTESIAN_POINT('Ctrl Pts',(42.0133312280121,263.,24.9836191849968)) ;
#101188=CARTESIAN_POINT('Ctrl Pts',(42.0095039151958,263.,25.0522555711132)) ;
#101189=CARTESIAN_POINT('Ctrl Pts',(42.001407309068,263.,25.1206549432494)) ;
#101190=CARTESIAN_POINT('Ctrl Pts',(41.9892161635851,263.,25.1885066891326)) ;
#101191=CARTESIAN_POINT('Ctrl Pts',(41.9834556365975,263.,25.2205678120075)) ;
#101192=CARTESIAN_POINT('Ctrl Pts',(41.9767802052095,263.,25.252506372225)) ;
#101193=CARTESIAN_POINT('Ctrl Pts',(41.9692048103826,263.,25.2842875802732)) ;
#101194=CARTESIAN_POINT('Ctrl Pts',(41.9661292099625,263.,25.2971907092924)) ;
#101195=CARTESIAN_POINT('Ctrl Pts',(41.9629052404632,263.,25.310067883192)) ;
#101196=CARTESIAN_POINT('Ctrl Pts',(41.9595338081523,263.,25.3229166948442)) ;
#101197=CARTESIAN_POINT('Ctrl Pts',(41.9566264007368,263.,25.3339970686539)) ;
#101198=CARTESIAN_POINT('Ctrl Pts',(41.9536092891766,263.,25.3450561348907)) ;
#101199=CARTESIAN_POINT('Ctrl Pts',(41.9504871902772,263.,25.3560786681579)) ;
#101200=CARTESIAN_POINT('Ctrl Pts',(41.9320746739268,263.,25.4210838395316)) ;
#101201=CARTESIAN_POINT('Ctrl Pts',(41.9099834503833,263.,25.484942222437)) ;
#101202=CARTESIAN_POINT('Ctrl Pts',(41.8844163316153,263.,25.5473739875613)) ;
#101203=CARTESIAN_POINT('Ctrl Pts',(41.8588447200449,263.,25.6098167235577)) ;
#101204=CARTESIAN_POINT('Ctrl Pts',(41.8297953520112,263.,25.6708332212835)) ;
#101205=CARTESIAN_POINT('Ctrl Pts',(41.7974260930702,263.,25.7301185903455)) ;
#101206=CARTESIAN_POINT('Ctrl Pts',(41.7652951541796,263.,25.7889674683475)) ;
#101207=CARTESIAN_POINT('Ctrl Pts',(41.7298923901342,263.,25.8461114160743)) ;
#101208=CARTESIAN_POINT('Ctrl Pts',(41.6913374251241,263.,25.9012152058858)) ;
#101209=CARTESIAN_POINT('Ctrl Pts',(41.6836283485783,263.,25.9122332247975)) ;
#101210=CARTESIAN_POINT('Ctrl Pts',(41.6757931522158,263.,25.9231695365843)) ;
#101211=CARTESIAN_POINT('Ctrl Pts',(41.667832658191,263.,25.9340212385773)) ;
#101212=CARTESIAN_POINT('Ctrl Pts',(41.660906427956,263.,25.9434630378188)) ;
#101213=CARTESIAN_POINT('Ctrl Pts',(41.6538848142978,263.,25.9528413248573)) ;
#101214=CARTESIAN_POINT('Ctrl Pts',(41.646778399557,263.,25.962141416589)) ;
#101215=CARTESIAN_POINT('Ctrl Pts',(41.6066123392045,263.,26.0147063258163)) ;
#101216=CARTESIAN_POINT('Ctrl Pts',(41.5636680906624,263.,26.0648760908122)) ;
#101217=CARTESIAN_POINT('Ctrl Pts',(41.5181015106568,263.,26.112369179746)) ;
#101218=CARTESIAN_POINT('Ctrl Pts',(41.4738500584133,263.,26.1584915386457)) ;
#101219=CARTESIAN_POINT('Ctrl Pts',(41.4271247588532,263.,26.2020900403433)) ;
#101220=CARTESIAN_POINT('Ctrl Pts',(41.3780390291705,263.,26.2428690423025)) ;
#101221=CARTESIAN_POINT('Ctrl Pts',(41.3294671498362,263.,26.2832211522811)) ;
#101222=CARTESIAN_POINT('Ctrl Pts',(41.278583472291,263.,26.3208130709105)) ;
#101223=CARTESIAN_POINT('Ctrl Pts',(41.2254776126781,263.,26.3553123614681)) ;
#101224=CARTESIAN_POINT('Ctrl Pts',(41.2086540352895,263.,26.3662415035399)) ;
#101225=CARTESIAN_POINT('Ctrl Pts',(41.1916073222241,263.,26.3768598912907)) ;
#101226=CARTESIAN_POINT('Ctrl Pts',(41.1743400212929,263.,26.3871558334365)) ;
#101227=CARTESIAN_POINT('',(39.2243975151537,262.999430917611,26.3874606005124)) ;
#101228=CARTESIAN_POINT('Ctrl Pts',(39.2427274574787,263.,26.3991716932468)) ;
#101229=CARTESIAN_POINT('Ctrl Pts',(39.2367806955717,262.99981030587,26.3950401358826)) ;
#101230=CARTESIAN_POINT('Ctrl Pts',(39.2308606815433,262.999620611741,26.3908700789342)) ;
#101231=CARTESIAN_POINT('Ctrl Pts',(39.2249679116208,262.999430917611,26.386661871944)) ;
#101232=CARTESIAN_POINT('Ctrl Pts',(39.2237775472856,263.,26.388236458444)) ;
#101233=CARTESIAN_POINT('Ctrl Pts',(39.1669376385685,263.,26.3549247848828)) ;
#101234=CARTESIAN_POINT('Ctrl Pts',(39.1123107922543,263.,26.3182679632608)) ;
#101235=CARTESIAN_POINT('Ctrl Pts',(39.0602509694005,263.,26.2783516922222)) ;
#101236=CARTESIAN_POINT('Ctrl Pts',(39.0544382172448,263.,26.2738948312917)) ;
#101237=CARTESIAN_POINT('Ctrl Pts',(39.0486574820743,263.,26.2693972834884)) ;
#101238=CARTESIAN_POINT('Ctrl Pts',(39.0429092691825,263.,26.264859129371)) ;
#101239=CARTESIAN_POINT('Ctrl Pts',(39.0082261335841,263.,26.2374771556025)) ;
#101240=CARTESIAN_POINT('Ctrl Pts',(38.974726487123,263.,26.2086177375078)) ;
#101241=CARTESIAN_POINT('Ctrl Pts',(38.9424340004638,263.,26.1783897705185)) ;
#101242=CARTESIAN_POINT('Ctrl Pts',(38.9236083074801,263.,26.1607676396474)) ;
#101243=CARTESIAN_POINT('Ctrl Pts',(38.9051929933829,263.,26.1426801918312)) ;
#101244=CARTESIAN_POINT('Ctrl Pts',(38.8871938087522,263.,26.1241474718767)) ;
#101245=CARTESIAN_POINT('Ctrl Pts',(38.8774589630145,263.,26.1141240639523)) ;
#101246=CARTESIAN_POINT('Ctrl Pts',(38.8678456247877,263.,26.1039699594861)) ;
#101247=CARTESIAN_POINT('Ctrl Pts',(38.8583651879793,263.,26.0936999832725)) ;
#101248=CARTESIAN_POINT('Ctrl Pts',(38.8138474201968,263.,26.0454747352747)) ;
#101249=CARTESIAN_POINT('Ctrl Pts',(38.7721995286391,263.,25.9946393686953)) ;
#101250=CARTESIAN_POINT('Ctrl Pts',(38.7334891808602,263.,25.9415526275785)) ;
#101251=CARTESIAN_POINT('Ctrl Pts',(38.7023688985965,263.,25.898874778817)) ;
#101252=CARTESIAN_POINT('Ctrl Pts',(38.673147542335,263.,25.8547406920465)) ;
#101253=CARTESIAN_POINT('Ctrl Pts',(38.645875368868,263.,25.8093176005942)) ;
#101254=CARTESIAN_POINT('Ctrl Pts',(38.6367093756936,263.,25.7940512065638)) ;
#101255=CARTESIAN_POINT('Ctrl Pts',(38.6277636836788,263.,25.7786390871617)) ;
#101256=CARTESIAN_POINT('Ctrl Pts',(38.6190405938922,263.,25.7630872526879)) ;
#101257=CARTESIAN_POINT('Ctrl Pts',(38.6116128714022,263.,25.7498448450654)) ;
#101258=CARTESIAN_POINT('Ctrl Pts',(38.6043456429172,263.,25.7364991203329)) ;
#101259=CARTESIAN_POINT('Ctrl Pts',(38.5972509227465,263.,25.7230744078097)) ;
#101260=CARTESIAN_POINT('Ctrl Pts',(38.5653661356432,263.,25.6627416405649)) ;
#101261=CARTESIAN_POINT('Ctrl Pts',(38.5369123809752,263.,25.6007297614524)) ;
#101262=CARTESIAN_POINT('Ctrl Pts',(38.5119644979003,263.,25.5374093499191)) ;
#101263=CARTESIAN_POINT('Ctrl Pts',(38.4870571409114,263.,25.4741917979528)) ;
#101264=CARTESIAN_POINT('Ctrl Pts',(38.465643799872,263.,25.4096690022917)) ;
#101265=CARTESIAN_POINT('Ctrl Pts',(38.447837750618,263.,25.3441753824993)) ;
#101266=CARTESIAN_POINT('Ctrl Pts',(38.4346381616535,263.,25.2956250921608)) ;
#101267=CARTESIAN_POINT('Ctrl Pts',(38.4234216189492,263.,25.2465405280528)) ;
#101268=CARTESIAN_POINT('Ctrl Pts',(38.414250442511,263.,25.1970504156763)) ;
#101269=CARTESIAN_POINT('Ctrl Pts',(38.4090270872937,263.,25.1688637987869)) ;
#101270=CARTESIAN_POINT('Ctrl Pts',(38.4044674641103,263.,25.140545538497)) ;
#101271=CARTESIAN_POINT('Ctrl Pts',(38.4005853285551,263.,25.1121189487793)) ;
#101272=CARTESIAN_POINT('Ctrl Pts',(38.3986277653732,263.,25.0977848678006)) ;
#101273=CARTESIAN_POINT('Ctrl Pts',(38.3968422492944,263.,25.0834199356196)) ;
#101274=CARTESIAN_POINT('Ctrl Pts',(38.3952331809663,263.,25.0690525878883)) ;
#101275=CARTESIAN_POINT('Ctrl Pts',(38.3874502671335,263.,24.9995590633116)) ;
#101276=CARTESIAN_POINT('Ctrl Pts',(38.3837740175701,263.,24.9298951051885)) ;
#101277=CARTESIAN_POINT('Ctrl Pts',(38.384311998664,263.,24.8604163963716)) ;
#101278=CARTESIAN_POINT('Ctrl Pts',(38.3846040717562,263.,24.8226959977267)) ;
#101279=CARTESIAN_POINT('Ctrl Pts',(38.3861390574197,263.,24.7850297485891)) ;
#101280=CARTESIAN_POINT('Ctrl Pts',(38.3889402251797,263.,24.7474723441793)) ;
#101281=CARTESIAN_POINT('Ctrl Pts',(38.3939657642221,263.,24.680091088087)) ;
#101282=CARTESIAN_POINT('Ctrl Pts',(38.4030636298359,263.,24.6130599957594)) ;
#101283=CARTESIAN_POINT('Ctrl Pts',(38.4160158840873,263.,24.5466214244428)) ;
#101284=CARTESIAN_POINT('Ctrl Pts',(38.422527882029,263.,24.51321813948)) ;
#101285=CARTESIAN_POINT('Ctrl Pts',(38.4300150165224,263.,24.4799646157873)) ;
#101286=CARTESIAN_POINT('Ctrl Pts',(38.4384544132907,263.,24.4468920772989)) ;
#101287=CARTESIAN_POINT('Ctrl Pts',(38.4425981998155,263.,24.4306532935215)) ;
#101288=CARTESIAN_POINT('Ctrl Pts',(38.4469716106731,263.,24.4144581511406)) ;
#101289=CARTESIAN_POINT('Ctrl Pts',(38.451572204719,263.,24.3983104098412)) ;
#101290=CARTESIAN_POINT('Ctrl Pts',(38.4544388118984,263.,24.3882488328627)) ;
#101291=CARTESIAN_POINT('Ctrl Pts',(38.4573929319971,263.,24.3782082726981)) ;
#101292=CARTESIAN_POINT('Ctrl Pts',(38.4604312466437,263.,24.368197766504)) ;
#101293=CARTESIAN_POINT('Ctrl Pts',(38.4806470280642,263.,24.3015916941675)) ;
#101294=CARTESIAN_POINT('Ctrl Pts',(38.5046153480752,263.,24.2362112258845)) ;
#101295=CARTESIAN_POINT('Ctrl Pts',(38.5320710142609,263.,24.1723085240421)) ;
#101296=CARTESIAN_POINT('Ctrl Pts',(38.5601590227769,263.,24.1069340537449)) ;
#101297=CARTESIAN_POINT('Ctrl Pts',(38.5918971212003,263.,24.0431053156208)) ;
#101298=CARTESIAN_POINT('Ctrl Pts',(38.6270568318401,263.,23.9810964403393)) ;
#101299=CARTESIAN_POINT('Ctrl Pts',(38.6621511208827,263.,23.9192029448372)) ;
#101300=CARTESIAN_POINT('Ctrl Pts',(38.700654786082,263.,23.8591216331877)) ;
#101301=CARTESIAN_POINT('Ctrl Pts',(38.742389300636,263.,23.8011427668039)) ;
#101302=CARTESIAN_POINT('Ctrl Pts',(38.7526688381686,263.,23.7868621182937)) ;
#101303=CARTESIAN_POINT('Ctrl Pts',(38.7631445953972,263.,23.7727091410837)) ;
#101304=CARTESIAN_POINT('Ctrl Pts',(38.7738143068348,263.,23.7586884371728)) ;
#101305=CARTESIAN_POINT('Ctrl Pts',(38.7824522458874,263.,23.7473376160596)) ;
#101306=CARTESIAN_POINT('Ctrl Pts',(38.7912188006332,263.,23.7360718015792)) ;
#101307=CARTESIAN_POINT('Ctrl Pts',(38.8000982758865,263.,23.7249112410076)) ;
#101308=CARTESIAN_POINT('Ctrl Pts',(38.8456525266383,263.,23.6676543693683)) ;
#101309=CARTESIAN_POINT('Ctrl Pts',(38.8942517906015,263.,23.6130628129694)) ;
#101310=CARTESIAN_POINT('Ctrl Pts',(38.9456535024128,263.,23.5614140617915)) ;
#101311=CARTESIAN_POINT('Ctrl Pts',(38.996702915142,263.,23.5101193028638)) ;
#101312=CARTESIAN_POINT('Ctrl Pts',(39.0505170528315,263.,23.4617262579711)) ;
#101313=CARTESIAN_POINT('Ctrl Pts',(39.1069036408252,263.,23.4165290640856)) ;
#101314=CARTESIAN_POINT('Ctrl Pts',(39.1626773094991,263.,23.3718231613798)) ;
#101315=CARTESIAN_POINT('Ctrl Pts',(39.2209683536167,263.,23.3302431739907)) ;
#101316=CARTESIAN_POINT('Ctrl Pts',(39.2816269746244,263.,23.2921084083525)) ;
#101317=CARTESIAN_POINT('Ctrl Pts',(39.3034799837762,263.,23.2783698932223)) ;
#101318=CARTESIAN_POINT('Ctrl Pts',(39.3256405828265,263.,23.2650789194409)) ;
#101319=CARTESIAN_POINT('Ctrl Pts',(39.3481027319428,263.,23.25225186137)) ;
#101320=CARTESIAN_POINT('Ctrl Pts',(40.9266772327442,265.16663141208,23.5122865229654)) ;
#101321=CARTESIAN_POINT('Ctrl Pts',(41.4154229970103,265.140857866373,23.7476426923537)) ;
#101322=CARTESIAN_POINT('Ctrl Pts',(42.139053620203,265.089310774958,24.7267012755206)) ;
#101323=CARTESIAN_POINT('Ctrl Pts',(41.537785195068,265.011990137836,26.4588392827834)) ;
#101324=CARTESIAN_POINT('Ctrl Pts',(39.767321066632,264.934669500713,26.9357152639846)) ;
#101325=CARTESIAN_POINT('Ctrl Pts',(38.3751878547293,264.857348863591,25.744116361454)) ;
#101326=CARTESIAN_POINT('Ctrl Pts',(38.5739887027783,264.780028226469,23.9217644529074)) ;
#101327=CARTESIAN_POINT('Ctrl Pts',(40.191063261612,264.702707589347,23.0585544040981)) ;
#101328=CARTESIAN_POINT('Ctrl Pts',(41.8158285227973,264.625386952225,23.9069987676438)) ;
#101329=CARTESIAN_POINT('Ctrl Pts',(42.0314636541983,264.548066315103,25.72729466396)) ;
#101330=CARTESIAN_POINT('Ctrl Pts',(40.6498435869966,264.47074567798,26.9318857254471)) ;
#101331=CARTESIAN_POINT('Ctrl Pts',(38.8759213080425,264.393425040858,26.4702669479006)) ;
#101332=CARTESIAN_POINT('Ctrl Pts',(38.2567337248227,264.316104403736,24.7450065743952)) ;
#101333=CARTESIAN_POINT('Ctrl Pts',(39.3322857677736,264.238783766614,23.2607234419196)) ;
#101334=CARTESIAN_POINT('Ctrl Pts',(41.1645770980241,264.161463129492,23.3118696438206)) ;
#101335=CARTESIAN_POINT('Ctrl Pts',(42.1556538103889,264.084142492369,24.8538413017259)) ;
#101336=CARTESIAN_POINT('Ctrl Pts',(41.4411893612298,264.006821855247,26.5418727571386)) ;
#101337=CARTESIAN_POINT('Ctrl Pts',(39.6442745448301,263.929501218125,26.9038183269182)) ;
#101338=CARTESIAN_POINT('Ctrl Pts',(38.3320113478042,263.852180581003,25.6240238449097)) ;
#101339=CARTESIAN_POINT('Ctrl Pts',(38.648837232223,263.774859943881,23.8186047859197)) ;
#101340=CARTESIAN_POINT('Ctrl Pts',(40.3184403474066,263.697539306759,23.0620880410149)) ;
#101341=CARTESIAN_POINT('Ctrl Pts',(41.8847589041631,263.620218669636,24.0142223877692)) ;
#101342=CARTESIAN_POINT('Ctrl Pts',(41.9817681831547,263.542898032514,25.8446772109839)) ;
#101343=CARTESIAN_POINT('Ctrl Pts',(40.5249220723503,263.465577395392,26.9570258080617)) ;
#101344=CARTESIAN_POINT('Ctrl Pts',(38.7846224372234,263.38825675827,26.381335876614)) ;
#101345=CARTESIAN_POINT('Ctrl Pts',(38.2788622298172,263.310936121148,24.6193214418341)) ;
#101346=CARTESIAN_POINT('Ctrl Pts',(39.448117170112,263.233615484025,23.2083693842535)) ;
#101347=CARTESIAN_POINT('Ctrl Pts',(41.2738845567306,263.156294846903,23.377269891905)) ;
#101348=CARTESIAN_POINT('Ctrl Pts',(42.1610135674441,263.078965437305,24.9821346196071)) ;
#101349=CARTESIAN_POINT('Ctrl Pts',(41.6141021871797,263.027409573415,26.0701640241726)) ;
#101350=CARTESIAN_POINT('Ctrl Pts',(41.1722257452137,263.001627255232,26.3851458267893)) ;
#101351=CARTESIAN_POINT('Ctrl Pts',(40.9687759254743,265.110610308119,23.4248634577175)) ;
#101352=CARTESIAN_POINT('Ctrl Pts',(41.4858362657664,265.084836762411,23.673854548651)) ;
#101353=CARTESIAN_POINT('Ctrl Pts',(42.2513890820361,265.033289670997,24.7096330682631)) ;
#101354=CARTESIAN_POINT('Ctrl Pts',(41.6152872899847,264.955969033874,26.542119266508)) ;
#101355=CARTESIAN_POINT('Ctrl Pts',(39.7422546180825,264.878648396752,27.0466221699495)) ;
#101356=CARTESIAN_POINT('Ctrl Pts',(38.2694707600797,264.80132775963,25.7859902032268)) ;
#101357=CARTESIAN_POINT('Ctrl Pts',(38.4797887651819,264.724007122508,23.8580637292653)) ;
#101358=CARTESIAN_POINT('Ctrl Pts',(40.1905455283097,264.646686485386,22.9448452131905)) ;
#101359=CARTESIAN_POINT('Ctrl Pts',(41.9094385403132,264.569365848263,23.8424426215131)) ;
#101360=CARTESIAN_POINT('Ctrl Pts',(42.1375660916355,264.492045211141,25.768193972003)) ;
#101361=CARTESIAN_POINT('Ctrl Pts',(40.6759044378011,264.414724574019,27.0425707742258)) ;
#101362=CARTESIAN_POINT('Ctrl Pts',(38.7992132738682,264.337403936897,26.5542089721305)) ;
#101363=CARTESIAN_POINT('Ctrl Pts',(38.1441542106657,264.260083299775,24.7289988505517)) ;
#101364=CARTESIAN_POINT('Ctrl Pts',(39.2820163590266,264.182762662652,23.1587265378696)) ;
#101365=CARTESIAN_POINT('Ctrl Pts',(41.2204580765855,264.10544202553,23.2128357997664)) ;
#101366=CARTESIAN_POINT('Ctrl Pts',(42.2689509733383,264.028121388408,24.8441387152086)) ;
#101367=CARTESIAN_POINT('Ctrl Pts',(41.5130953563313,263.950800751286,26.6299631306286)) ;
#101368=CARTESIAN_POINT('Ctrl Pts',(39.6120796250978,263.873480114164,27.0128773432121)) ;
#101369=CARTESIAN_POINT('Ctrl Pts',(38.2237929026015,263.796159477042,25.6589403502952)) ;
#101370=CARTESIAN_POINT('Ctrl Pts',(38.5589735048453,263.718838839919,23.7489276990081)) ;
#101371=CARTESIAN_POINT('Ctrl Pts',(40.3253019684505,263.641518202797,22.948583564784)) ;
#101372=CARTESIAN_POINT('Ctrl Pts',(41.9823622750059,263.564197565675,23.9558780424679)) ;
#101373=CARTESIAN_POINT('Ctrl Pts',(42.0849916059877,263.486876928553,25.8923768583746)) ;
#101374=CARTESIAN_POINT('Ctrl Pts',(40.5437458277518,263.409556291431,27.069167300727)) ;
#101375=CARTESIAN_POINT('Ctrl Pts',(38.702625172926,263.332235654309,26.460125844779)) ;
#101376=CARTESIAN_POINT('Ctrl Pts',(38.1675646894037,263.254915017186,24.5960323838054)) ;
#101377=CARTESIAN_POINT('Ctrl Pts',(39.4045582380329,263.177594380064,23.1033394453326)) ;
#101378=CARTESIAN_POINT('Ctrl Pts',(41.3360980594305,263.100273742942,23.2820248894775)) ;
#101379=CARTESIAN_POINT('Ctrl Pts',(42.2746212379409,263.022944333345,24.9798644676362)) ;
#101380=CARTESIAN_POINT('Ctrl Pts',(41.696025564966,262.971388469454,26.1309268303295)) ;
#101381=CARTESIAN_POINT('Ctrl Pts',(41.2285498339117,262.945606151272,26.4641565173252)) ;
#101382=CARTESIAN_POINT('Ctrl Pts',(41.0108746182042,265.054589204158,23.3374403924696)) ;
#101383=CARTESIAN_POINT('Ctrl Pts',(41.5562495345224,265.028815658451,23.6000664049484)) ;
#101384=CARTESIAN_POINT('Ctrl Pts',(42.3637245438692,264.977268567036,24.6925648610056)) ;
#101385=CARTESIAN_POINT('Ctrl Pts',(41.6927893849013,264.899947929914,26.6253992502325)) ;
#101386=CARTESIAN_POINT('Ctrl Pts',(39.7171881695331,264.822627292792,27.1575290759145)) ;
#101387=CARTESIAN_POINT('Ctrl Pts',(38.1637536654301,264.74530665567,25.8278640449995)) ;
#101388=CARTESIAN_POINT('Ctrl Pts',(38.3855888275855,264.667986018547,23.7943630056233)) ;
#101389=CARTESIAN_POINT('Ctrl Pts',(40.1900277950074,264.590665381425,22.8311360222829)) ;
#101390=CARTESIAN_POINT('Ctrl Pts',(42.0030485578291,264.513344744303,23.7778864753824)) ;
#101391=CARTESIAN_POINT('Ctrl Pts',(42.2436685290726,264.436024107181,25.8090932800459)) ;
#101392=CARTESIAN_POINT('Ctrl Pts',(40.7019652886055,264.358703470059,27.1532558230045)) ;
#101393=CARTESIAN_POINT('Ctrl Pts',(38.7225052396939,264.281382832936,26.6381509963604)) ;
#101394=CARTESIAN_POINT('Ctrl Pts',(38.0315746965087,264.204062195814,24.7129911267082)) ;
#101395=CARTESIAN_POINT('Ctrl Pts',(39.2317469502797,264.126741558692,23.0567296338196)) ;
#101396=CARTESIAN_POINT('Ctrl Pts',(41.276339055147,264.04942092157,23.113801955712)) ;
#101397=CARTESIAN_POINT('Ctrl Pts',(42.3822481362876,263.972100284448,24.8344361286912)) ;
#101398=CARTESIAN_POINT('Ctrl Pts',(41.585001351433,263.894779647326,26.7180535041185)) ;
#101399=CARTESIAN_POINT('Ctrl Pts',(39.5798847053656,263.817459010204,27.121936359506)) ;
#101400=CARTESIAN_POINT('Ctrl Pts',(38.1155744573986,263.740138373081,25.6938568556807)) ;
#101401=CARTESIAN_POINT('Ctrl Pts',(38.4691097774677,263.662817735959,23.6792506120963)) ;
#101402=CARTESIAN_POINT('Ctrl Pts',(40.3321635894945,263.585497098837,22.8350790885532)) ;
#101403=CARTESIAN_POINT('Ctrl Pts',(42.0799656458485,263.508176461715,23.8975336971666)) ;
#101404=CARTESIAN_POINT('Ctrl Pts',(42.1882150288208,263.430855824592,25.9400765057655)) ;
#101405=CARTESIAN_POINT('Ctrl Pts',(40.5625695831534,263.35353518747,27.1813087933923)) ;
#101406=CARTESIAN_POINT('Ctrl Pts',(38.6206279086286,263.276214550348,26.5389158129438)) ;
#101407=CARTESIAN_POINT('Ctrl Pts',(38.0562671489902,263.198893913226,24.5727433257766)) ;
#101408=CARTESIAN_POINT('Ctrl Pts',(39.360999305954,263.121573276104,22.9983095064116)) ;
#101409=CARTESIAN_POINT('Ctrl Pts',(41.3983115621305,263.044252638982,23.1867798870499)) ;
#101410=CARTESIAN_POINT('Ctrl Pts',(42.3882289084377,262.966923229383,24.9775943156654)) ;
#101411=CARTESIAN_POINT('Ctrl Pts',(41.7779489427525,262.915367365494,26.1916896364865)) ;
#101412=CARTESIAN_POINT('Ctrl Pts',(41.2848739226097,262.889585047311,26.543167207861)) ;
#101413=CARTESIAN_POINT('Ctrl Pts',(41.0529733109342,264.998568100198,23.2500173272218)) ;
#101414=CARTESIAN_POINT('Ctrl Pts',(41.6266628032785,264.972794554491,23.5262782612457)) ;
#101415=CARTESIAN_POINT('Ctrl Pts',(42.4760600057023,264.921247463076,24.6754966537481)) ;
#101416=CARTESIAN_POINT('Ctrl Pts',(41.770291479818,264.843926825954,26.708679233957)) ;
#101417=CARTESIAN_POINT('Ctrl Pts',(39.6921217209837,264.766606188831,27.2684359818795)) ;
#101418=CARTESIAN_POINT('Ctrl Pts',(38.0580365707805,264.689285551709,25.8697378867723)) ;
#101419=CARTESIAN_POINT('Ctrl Pts',(38.291388889989,264.611964914587,23.7306622819812)) ;
#101420=CARTESIAN_POINT('Ctrl Pts',(40.1895100617051,264.534644277465,22.7174268313754)) ;
#101421=CARTESIAN_POINT('Ctrl Pts',(42.096658575345,264.457323640343,23.7133303292517)) ;
#101422=CARTESIAN_POINT('Ctrl Pts',(42.3497709665098,264.38000300322,25.8499925880888)) ;
#101423=CARTESIAN_POINT('Ctrl Pts',(40.7280261394099,264.302682366099,27.2639408717831)) ;
#101424=CARTESIAN_POINT('Ctrl Pts',(38.6457972055196,264.225361728976,26.7220930205903)) ;
#101425=CARTESIAN_POINT('Ctrl Pts',(37.9189951823518,264.148041091854,24.6969834028647)) ;
#101426=CARTESIAN_POINT('Ctrl Pts',(39.1814775415326,264.070720454732,22.9547327297695)) ;
#101427=CARTESIAN_POINT('Ctrl Pts',(41.3322200337085,263.99339981761,23.0147681116578)) ;
#101428=CARTESIAN_POINT('Ctrl Pts',(42.4955452992371,263.916079180488,24.8247335421739)) ;
#101429=CARTESIAN_POINT('Ctrl Pts',(41.6569073465345,263.838758543365,26.8061438776086)) ;
#101430=CARTESIAN_POINT('Ctrl Pts',(39.5476897856333,263.761437906243,27.2309953757999)) ;
#101431=CARTESIAN_POINT('Ctrl Pts',(38.0073560121957,263.684117269121,25.7287733610662)) ;
#101432=CARTESIAN_POINT('Ctrl Pts',(38.37924605009,263.606796631999,23.6095735251847)) ;
#101433=CARTESIAN_POINT('Ctrl Pts',(40.3390252105383,263.529475994877,22.7215746123224)) ;
#101434=CARTESIAN_POINT('Ctrl Pts',(42.1775690166913,263.452155357755,23.8391893518654)) ;
#101435=CARTESIAN_POINT('Ctrl Pts',(42.2914384516538,263.374834720632,25.9877761531562)) ;
#101436=CARTESIAN_POINT('Ctrl Pts',(40.5813933385549,263.29751408351,27.2934502860576)) ;
#101437=CARTESIAN_POINT('Ctrl Pts',(38.5386306443311,263.220193446388,26.6177057811087)) ;
#101438=CARTESIAN_POINT('Ctrl Pts',(37.9449696085767,263.142872809266,24.5494542677479)) ;
#101439=CARTESIAN_POINT('Ctrl Pts',(39.3174403738751,263.065552172143,22.8932795674907)) ;
#101440=CARTESIAN_POINT('Ctrl Pts',(41.4605250648304,262.988231535021,23.0915348846222)) ;
#101441=CARTESIAN_POINT('Ctrl Pts',(42.5018365789347,262.910902125423,24.9753241636946)) ;
#101442=CARTESIAN_POINT('Ctrl Pts',(41.859872320539,262.859346261533,26.2524524426436)) ;
#101443=CARTESIAN_POINT('Ctrl Pts',(41.3411980113077,262.83356394335,26.6221778983969)) ;
#101444=CARTESIAN_POINT('',(41.1755994881009,265.000571825747,26.3874569216172)) ;
#101445=CARTESIAN_POINT('Ctrl Pts',(41.176222444591,265.,26.3882365197604)) ;
#101446=CARTESIAN_POINT('Ctrl Pts',(41.2333448641361,265.,26.3547592787871)) ;
#101447=CARTESIAN_POINT('Ctrl Pts',(41.2881836897428,265.,26.3179317509912)) ;
#101448=CARTESIAN_POINT('Ctrl Pts',(41.3403904534507,265.,26.2778596828438)) ;
#101449=CARTESIAN_POINT('Ctrl Pts',(41.345987616831,265.,26.2735634978962)) ;
#101450=CARTESIAN_POINT('Ctrl Pts',(41.3515545184604,265.,26.2692299705254)) ;
#101451=CARTESIAN_POINT('Ctrl Pts',(41.3570907214659,265.,26.2648591961635)) ;
#101452=CARTESIAN_POINT('Ctrl Pts',(41.4074661306217,265.,26.2250883375815)) ;
#101453=CARTESIAN_POINT('Ctrl Pts',(41.455301981662,265.,26.1822376146413)) ;
#101454=CARTESIAN_POINT('Ctrl Pts',(41.5005335798205,265.,26.136649754872)) ;
#101455=CARTESIAN_POINT('Ctrl Pts',(41.5445252571308,265.,26.0923115820485)) ;
#101456=CARTESIAN_POINT('Ctrl Pts',(41.5860537828374,265.,26.0453833811781)) ;
#101457=CARTESIAN_POINT('Ctrl Pts',(41.6250320641521,265.,25.9961420649553)) ;
#101458=CARTESIAN_POINT('Ctrl Pts',(41.6367111946857,265.,25.9813878033404)) ;
#101459=CARTESIAN_POINT('Ctrl Pts',(41.6481611587152,265.,25.9664256536038)) ;
#101460=CARTESIAN_POINT('Ctrl Pts',(41.6593790545329,265.,25.9512625482557)) ;
#101461=CARTESIAN_POINT('Ctrl Pts',(41.6666618959751,265.,25.9414184122595)) ;
#101462=CARTESIAN_POINT('Ctrl Pts',(41.6738419690629,265.,25.9314961857445)) ;
#101463=CARTESIAN_POINT('Ctrl Pts',(41.6809150430192,265.,25.9215036288907)) ;
#101464=CARTESIAN_POINT('Ctrl Pts',(41.7192968173398,265.,25.8672793885651)) ;
#101465=CARTESIAN_POINT('Ctrl Pts',(41.754566870104,265.,25.8109384347298)) ;
#101466=CARTESIAN_POINT('Ctrl Pts',(41.7866620719983,265.,25.7528431024233)) ;
#101467=CARTESIAN_POINT('Ctrl Pts',(41.8200023630589,265.,25.6924940416903)) ;
#101468=CARTESIAN_POINT('Ctrl Pts',(41.8499174491227,265.,25.6302511300383)) ;
#101469=CARTESIAN_POINT('Ctrl Pts',(41.8762982392818,265.,25.5664770087076)) ;
#101470=CARTESIAN_POINT('Ctrl Pts',(41.902679029441,265.,25.5027028873769)) ;
#101471=CARTESIAN_POINT('Ctrl Pts',(41.9255260936111,265.,25.437396500668)) ;
#101472=CARTESIAN_POINT('Ctrl Pts',(41.9446830446594,265.,25.3708916870739)) ;
#101473=CARTESIAN_POINT('Ctrl Pts',(41.9479520979212,265.,25.3595429198689)) ;
#101474=CARTESIAN_POINT('Ctrl Pts',(41.951113571739,265.,25.3481592086006)) ;
#101475=CARTESIAN_POINT('Ctrl Pts',(41.9541665323496,265.,25.336742163306)) ;
#101476=CARTESIAN_POINT('Ctrl Pts',(41.9572422469794,265.,25.3252400256368)) ;
#101477=CARTESIAN_POINT('Ctrl Pts',(41.9602053850662,265.,25.3137130896354)) ;
#101478=CARTESIAN_POINT('Ctrl Pts',(41.9630546829663,265.,25.302166601324)) ;
#101479=CARTESIAN_POINT('Ctrl Pts',(41.9797320778241,265.,25.234583164443)) ;
#101480=CARTESIAN_POINT('Ctrl Pts',(41.9925227683547,265.,25.1662952212329)) ;
#101481=CARTESIAN_POINT('Ctrl Pts',(42.0013291177796,265.,25.0976636106023)) ;
#101482=CARTESIAN_POINT('Ctrl Pts',(42.0100463535875,265.,25.0297265001288)) ;
#101483=CARTESIAN_POINT('Ctrl Pts',(42.0148598907095,265.,24.9614516185098)) ;
#101484=CARTESIAN_POINT('Ctrl Pts',(42.0156297848673,265.,24.8931674279836)) ;
#101485=CARTESIAN_POINT('Ctrl Pts',(42.0161777252074,265.,24.8445689781833)) ;
#101486=CARTESIAN_POINT('Ctrl Pts',(42.0146765242096,265.,24.7959653337813)) ;
#101487=CARTESIAN_POINT('Ctrl Pts',(42.0110597486091,265.,24.7474724446513)) ;
#101488=CARTESIAN_POINT('Ctrl Pts',(42.0088703040113,265.,24.7181168788469)) ;
#101489=CARTESIAN_POINT('Ctrl Pts',(42.0059053067813,265.,24.6888018815549)) ;
#101490=CARTESIAN_POINT('Ctrl Pts',(42.0021799342865,265.,24.6595474945815)) ;
#101491=CARTESIAN_POINT('Ctrl Pts',(42.000315561177,265.,24.6449070546031)) ;
#101492=CARTESIAN_POINT('Ctrl Pts',(41.9982600471454,265.,24.6302782900132)) ;
#101493=CARTESIAN_POINT('Ctrl Pts',(41.9960195175212,265.,24.6156897113619)) ;
#101494=CARTESIAN_POINT('Ctrl Pts',(41.9858207846444,265.,24.5492835299357)) ;
#101495=CARTESIAN_POINT('Ctrl Pts',(41.9717814071419,265.,24.4836067190368)) ;
#101496=CARTESIAN_POINT('Ctrl Pts',(41.954161865892,265.,24.4188935223847)) ;
#101497=CARTESIAN_POINT('Ctrl Pts',(41.9358505721337,265.,24.3516396514054)) ;
#101498=CARTESIAN_POINT('Ctrl Pts',(41.9136724116091,265.,24.2854257589243)) ;
#101499=CARTESIAN_POINT('Ctrl Pts',(41.8878637011264,265.,24.2205124747507)) ;
#101500=CARTESIAN_POINT('Ctrl Pts',(41.8679078478126,265.,24.1703201190361)) ;
#101501=CARTESIAN_POINT('Ctrl Pts',(41.8457801865645,265.,24.1209051901021)) ;
#101502=CARTESIAN_POINT('Ctrl Pts',(41.8215690313579,265.,24.0723920420978)) ;
#101503=CARTESIAN_POINT('Ctrl Pts',(41.8084721454918,265.,24.0461491322906)) ;
#101504=CARTESIAN_POINT('Ctrl Pts',(41.7947652847443,265.,24.0201701869716)) ;
#101505=CARTESIAN_POINT('Ctrl Pts',(41.7804604108832,265.,23.9944757207669)) ;
#101506=CARTESIAN_POINT('Ctrl Pts',(41.7739393210212,265.,23.9827625155542)) ;
#101507=CARTESIAN_POINT('Ctrl Pts',(41.7672931345761,265.,23.971107065469)) ;
#101508=CARTESIAN_POINT('Ctrl Pts',(41.760525403896,265.,23.9595156589188)) ;
#101509=CARTESIAN_POINT('Ctrl Pts',(41.7240227911903,265.,23.8969959393823)) ;
#101510=CARTESIAN_POINT('Ctrl Pts',(41.6841159271636,265.,23.8365546621805)) ;
#101511=CARTESIAN_POINT('Ctrl Pts',(41.6410467668449,265.,23.778471424062)) ;
#101512=CARTESIAN_POINT('Ctrl Pts',(41.6017019158626,265.,23.7254108040865)) ;
#101513=CARTESIAN_POINT('Ctrl Pts',(41.5597171036843,265.,23.6743175785997)) ;
#101514=CARTESIAN_POINT('Ctrl Pts',(41.5152413929121,265.,23.6254187090586)) ;
#101515=CARTESIAN_POINT('Ctrl Pts',(41.5020529827085,265.,23.6109186968318)) ;
#101516=CARTESIAN_POINT('Ctrl Pts',(41.4886453392958,265.,23.5966117579114)) ;
#101517=CARTESIAN_POINT('Ctrl Pts',(41.4750218437445,265.,23.582504157239)) ;
#101518=CARTESIAN_POINT('Ctrl Pts',(41.4619489946405,265.,23.5689667700012)) ;
#101519=CARTESIAN_POINT('Ctrl Pts',(41.44867445627,265.,23.555610276238)) ;
#101520=CARTESIAN_POINT('Ctrl Pts',(41.4352209361124,265.,23.5424592086853)) ;
#101521=CARTESIAN_POINT('Ctrl Pts',(41.382909570539,265.,23.4913238705454)) ;
#101522=CARTESIAN_POINT('Ctrl Pts',(41.3278436810974,265.,23.4432360534943)) ;
#101523=CARTESIAN_POINT('Ctrl Pts',(41.2702341795315,265.,23.3984890066187)) ;
#101524=CARTESIAN_POINT('Ctrl Pts',(41.2131253011062,265.,23.3541308089176)) ;
#101525=CARTESIAN_POINT('Ctrl Pts',(41.1535162684096,265.,23.3130547011252)) ;
#101526=CARTESIAN_POINT('Ctrl Pts',(41.09157380261,265.,23.275578834956)) ;
#101527=CARTESIAN_POINT('Ctrl Pts',(41.0784526521616,265.,23.2676403960862)) ;
#101528=CARTESIAN_POINT('Ctrl Pts',(41.0652266755638,265.,23.2598636479025)) ;
#101529=CARTESIAN_POINT('Ctrl Pts',(41.0518972680585,265.,23.2522518613707)) ;
#101530=CARTESIAN_POINT('Ctrl Pts',(41.1750318437943,265.000571825747,26.3866620466095)) ;
#101531=CARTESIAN_POINT('Ctrl Pts',(41.1691390078094,265.000381217165,26.390870299183)) ;
#101532=CARTESIAN_POINT('Ctrl Pts',(41.1632189271215,265.000190608582,26.3950404008641)) ;
#101533=CARTESIAN_POINT('Ctrl Pts',(41.1572720979745,265.,26.3991720020989)) ;
#101534=CARTESIAN_POINT('Ctrl Pts',(39.0589035087791,265.166342823321,26.6220511683743)) ;
#101535=CARTESIAN_POINT('Ctrl Pts',(38.5402676181004,265.140560382316,26.2523570027814)) ;
#101536=CARTESIAN_POINT('Ctrl Pts',(37.8983515099597,265.089004395602,24.975331106744)) ;
#101537=CARTESIAN_POINT('Ctrl Pts',(38.9395788746228,265.011674863182,23.091694078747)) ;
#101538=CARTESIAN_POINT('Ctrl Pts',(41.0824868151442,264.934354226059,22.8934551200483)) ;
#101539=CARTESIAN_POINT('Ctrl Pts',(42.4548443959838,264.857033588937,24.5494931875868)) ;
#101540=CARTESIAN_POINT('Ctrl Pts',(41.8612323265555,264.779712951815,26.6175741202223)) ;
#101541=CARTESIAN_POINT('Ctrl Pts',(39.8186381174926,264.702392314693,27.2932628837251)) ;
#101542=CARTESIAN_POINT('Ctrl Pts',(38.108734046545,264.625071677571,25.9876964426934)) ;
#101543=CARTESIAN_POINT('Ctrl Pts',(38.2225940897709,264.547751040449,23.8392868516985)) ;
#101544=CARTESIAN_POINT('Ctrl Pts',(40.060986256048,264.470430403326,22.7217642917497)) ;
#101545=CARTESIAN_POINT('Ctrl Pts',(42.0206037771449,264.393109766204,23.609689963601)) ;
#101546=CARTESIAN_POINT('Ctrl Pts',(42.3924631422109,264.315789129082,25.7287150115834)) ;
#101547=CARTESIAN_POINT('Ctrl Pts',(40.8522564129019,264.23846849196,27.2308131254801)) ;
#101548=CARTESIAN_POINT('Ctrl Pts',(38.7432128167474,264.161147854838,26.805996668361)) ;
#101549=CARTESIAN_POINT('Ctrl Pts',(37.9046440334904,264.083827217716,24.8247497563215)) ;
#101550=CARTESIAN_POINT('Ctrl Pts',(39.0678733499127,264.006506580593,23.0149336087157)) ;
#101551=CARTESIAN_POINT('Ctrl Pts',(41.2184384524299,263.929185943471,22.9549031784783)) ;
#101552=CARTESIAN_POINT('Ctrl Pts',(42.4808166842117,263.851865306349,24.6970101535819)) ;
#101553=CARTESIAN_POINT('Ctrl Pts',(41.7540746063891,263.774544669227,26.7219527438018)) ;
#101554=CARTESIAN_POINT('Ctrl Pts',(39.6720174113598,263.697224032105,27.2637559039529)) ;
#101555=CARTESIAN_POINT('Ctrl Pts',(38.0504063428213,263.619903394982,25.849924240912)) ;
#101556=CARTESIAN_POINT('Ctrl Pts',(38.3034978579432,263.54258275786,23.7134382088736)) ;
#101557=CARTESIAN_POINT('Ctrl Pts',(40.2104890723333,263.465262120738,22.7176168533932)) ;
#101558=CARTESIAN_POINT('Ctrl Pts',(42.1084536899185,263.387941483616,23.7307687267153)) ;
#101559=CARTESIAN_POINT('Ctrl Pts',(42.3417867596045,263.310620846494,25.8696679088864)) ;
#101560=CARTESIAN_POINT('Ctrl Pts',(40.7078363774025,263.233300209372,27.2682506055213)) ;
#101561=CARTESIAN_POINT('Ctrl Pts',(38.6298380139055,263.155979572249,26.7085400306708)) ;
#101562=CARTESIAN_POINT('Ctrl Pts',(37.9241276393564,263.078658935127,24.67552500292)) ;
#101563=CARTESIAN_POINT('Ctrl Pts',(38.7734548453959,263.027111843712,23.5264015487631)) ;
#101564=CARTESIAN_POINT('Ctrl Pts',(39.3470970288687,263.001338298005,23.2501633963894)) ;
#101565=CARTESIAN_POINT('Ctrl Pts',(39.1152036213646,265.110345202765,26.543073337534)) ;
#101566=CARTESIAN_POINT('Ctrl Pts',(38.622156503643,265.084562761759,26.1916193674943)) ;
#101567=CARTESIAN_POINT('Ctrl Pts',(38.0119116427954,265.033006775045,24.9776001516761)) ;
#101568=CARTESIAN_POINT('Ctrl Pts',(39.0017662985697,264.955677242625,23.1868991528075)) ;
#101569=CARTESIAN_POINT('Ctrl Pts',(41.0389461440178,264.878356605503,22.9984410284024)) ;
#101570=CARTESIAN_POINT('Ctrl Pts',(42.3435935120022,264.801035968381,24.5727724827267)) ;
#101571=CARTESIAN_POINT('Ctrl Pts',(41.7792694358313,264.723715331259,26.5388171807061)) ;
#101572=CARTESIAN_POINT('Ctrl Pts',(39.8374539819582,264.646394694136,27.1811684011086)) ;
#101573=CARTESIAN_POINT('Ctrl Pts',(38.2119141978569,264.569074057014,25.9400167910603)) ;
#101574=CARTESIAN_POINT('Ctrl Pts',(38.3201565450318,264.491753419892,23.8976067389154)) ;
#101575=CARTESIAN_POINT('Ctrl Pts',(40.0678450006814,264.41443278277,22.8352211865956)) ;
#101576=CARTESIAN_POINT('Ctrl Pts',(41.9307777208776,264.337112145648,23.6793378417008)) ;
#101577=CARTESIAN_POINT('Ctrl Pts',(42.284290062462,264.259791508526,25.6938131432853)) ;
#101578=CARTESIAN_POINT('Ctrl Pts',(40.8200749893644,264.182470871404,27.1217998270116)) ;
#101579=CARTESIAN_POINT('Ctrl Pts',(38.8150886686681,264.105150234281,26.717943222585)) ;
#101580=CARTESIAN_POINT('Ctrl Pts',(38.0178937019737,264.027829597159,24.8344482754894)) ;
#101581=CARTESIAN_POINT('Ctrl Pts',(39.1237309030217,263.950508960037,23.1139259375247)) ;
#101582=CARTESIAN_POINT('Ctrl Pts',(41.1681901167507,263.873188322915,23.0568573251589)) ;
#101583=CARTESIAN_POINT('Ctrl Pts',(42.3682843636796,263.795867685793,24.7130111669482)) ;
#101584=CARTESIAN_POINT('Ctrl Pts',(41.6773987284251,263.71854704867,26.6380459082828)) ;
#101585=CARTESIAN_POINT('Ctrl Pts',(39.6980673373848,263.641226411548,27.1531172546474)) ;
#101586=CARTESIAN_POINT('Ctrl Pts',(38.1564643018487,263.563905774426,25.8090420779498)) ;
#101587=CARTESIAN_POINT('Ctrl Pts',(38.3970686338924,263.486585137304,23.7779672929588)) ;
#101588=CARTESIAN_POINT('Ctrl Pts',(40.2099715561041,263.409264500182,22.8312783770749)) ;
#101589=CARTESIAN_POINT('Ctrl Pts',(42.0142932412332,263.33194386306,23.7944427471727)) ;
#101590=CARTESIAN_POINT('Ctrl Pts',(42.236113982037,263.254623225937,25.8278116208275)) ;
#101591=CARTESIAN_POINT('Ctrl Pts',(40.6827804373985,263.177302588815,27.1573901938967)) ;
#101592=CARTESIAN_POINT('Ctrl Pts',(38.707307620792,263.099981951693,26.6252949597485)) ;
#101593=CARTESIAN_POINT('Ctrl Pts',(38.0364160138455,263.022661314571,24.6925860637149)) ;
#101594=CARTESIAN_POINT('Ctrl Pts',(38.843838597717,262.971114223156,23.600158761322)) ;
#101595=CARTESIAN_POINT('Ctrl Pts',(39.3891780743093,262.945340677449,23.3375498148907)) ;
#101596=CARTESIAN_POINT('Ctrl Pts',(39.1715037339501,265.054347582208,26.4640955066937)) ;
#101597=CARTESIAN_POINT('Ctrl Pts',(38.7040453891857,265.028565141203,26.1308817322073)) ;
#101598=CARTESIAN_POINT('Ctrl Pts',(38.1254717756312,264.977009154489,24.9798691966081)) ;
#101599=CARTESIAN_POINT('Ctrl Pts',(39.0639537225165,264.899679622069,23.282104226868)) ;
#101600=CARTESIAN_POINT('Ctrl Pts',(40.9954054728912,264.822358984947,23.1034269367565)) ;
#101601=CARTESIAN_POINT('Ctrl Pts',(42.2323426280205,264.745038347824,24.5960517778666)) ;
#101602=CARTESIAN_POINT('Ctrl Pts',(41.6973065451071,264.667717710702,26.4600602411901)) ;
#101603=CARTESIAN_POINT('Ctrl Pts',(39.8562698464239,264.59039707358,27.0690739184919)) ;
#101604=CARTESIAN_POINT('Ctrl Pts',(38.3150943491689,264.513076436458,25.8923371394272)) ;
#101605=CARTESIAN_POINT('Ctrl Pts',(38.4177190002927,264.435755799336,23.9559266261323)) ;
#101606=CARTESIAN_POINT('Ctrl Pts',(40.0747037453149,264.358435162214,22.9486780814416)) ;
#101607=CARTESIAN_POINT('Ctrl Pts',(41.8409516646104,264.281114525091,23.7489857198008)) ;
#101608=CARTESIAN_POINT('Ctrl Pts',(42.1761169827131,264.203793887969,25.6589112749871)) ;
#101609=CARTESIAN_POINT('Ctrl Pts',(40.7878935658271,264.126473250847,27.0127865285429)) ;
#101610=CARTESIAN_POINT('Ctrl Pts',(38.8869645205888,264.049152613725,26.6298897768089)) ;
#101611=CARTESIAN_POINT('Ctrl Pts',(38.131143370457,263.971831976603,24.8441467946573)) ;
#101612=CARTESIAN_POINT('Ctrl Pts',(39.1795884561308,263.894511339481,23.2129182663338)) ;
#101613=CARTESIAN_POINT('Ctrl Pts',(41.1179417810716,263.817190702358,23.1588114718395)) ;
#101614=CARTESIAN_POINT('Ctrl Pts',(42.2557520431477,263.739870065236,24.7290121803146)) ;
#101615=CARTESIAN_POINT('Ctrl Pts',(41.6007228504612,263.662549428114,26.5541390727638)) ;
#101616=CARTESIAN_POINT('Ctrl Pts',(39.7241172634097,263.585228790992,27.042478605342)) ;
#101617=CARTESIAN_POINT('Ctrl Pts',(38.2625222608762,263.50790815387,25.7681599149875)) ;
#101618=CARTESIAN_POINT('Ctrl Pts',(38.4906394098416,263.430587516748,23.842496377044)) ;
#101619=CARTESIAN_POINT('Ctrl Pts',(40.209454039875,263.353266879625,22.9449399007565)) ;
#101620=CARTESIAN_POINT('Ctrl Pts',(41.9201327925478,263.275946242503,23.8581167676299)) ;
#101621=CARTESIAN_POINT('Ctrl Pts',(42.1304412044695,263.198625605381,25.7859553327686)) ;
#101622=CARTESIAN_POINT('Ctrl Pts',(40.6577244973945,263.121304968259,27.046529782272)) ;
#101623=CARTESIAN_POINT('Ctrl Pts',(38.7847772276786,263.043984331137,26.5420498888262)) ;
#101624=CARTESIAN_POINT('Ctrl Pts',(38.1487043883347,262.966663694015,24.7096471245099)) ;
#101625=CARTESIAN_POINT('Ctrl Pts',(38.9142223500379,262.9151166026,23.673915973881)) ;
#101626=CARTESIAN_POINT('Ctrl Pts',(39.4312591197499,262.889343056892,23.424936233392)) ;
#101627=CARTESIAN_POINT('Ctrl Pts',(39.2278038465356,264.998349961652,26.3851176758534)) ;
#101628=CARTESIAN_POINT('Ctrl Pts',(38.7859342747284,264.972567520647,26.0701440969204)) ;
#101629=CARTESIAN_POINT('Ctrl Pts',(38.239031908467,264.921011533933,24.9821382415402)) ;
#101630=CARTESIAN_POINT('Ctrl Pts',(39.1261411464635,264.843682001513,23.3773093009285)) ;
#101631=CARTESIAN_POINT('Ctrl Pts',(40.9518648017648,264.76636136439,23.2084128451104)) ;
#101632=CARTESIAN_POINT('Ctrl Pts',(42.1210917440389,264.689040727268,24.6193310730064)) ;
#101633=CARTESIAN_POINT('Ctrl Pts',(41.6153436543828,264.611720090146,26.3813033016739)) ;
#101634=CARTESIAN_POINT('Ctrl Pts',(39.8750857108895,264.534399453024,26.9569794358752)) ;
#101635=CARTESIAN_POINT('Ctrl Pts',(38.4182745004808,264.457078815902,25.8446574877941)) ;
#101636=CARTESIAN_POINT('Ctrl Pts',(38.5152814555536,264.379758178779,24.0142465133491)) ;
#101637=CARTESIAN_POINT('Ctrl Pts',(40.0815624899484,264.302437541657,23.0621349762875)) ;
#101638=CARTESIAN_POINT('Ctrl Pts',(41.751125608343,264.225116904535,23.8186335979007)) ;
#101639=CARTESIAN_POINT('Ctrl Pts',(42.0679439029642,264.147796267413,25.6240094066889)) ;
#101640=CARTESIAN_POINT('Ctrl Pts',(40.7557121422897,264.070475630291,26.9037732300743)) ;
#101641=CARTESIAN_POINT('Ctrl Pts',(38.9588403725095,263.993154993169,26.5418363310329)) ;
#101642=CARTESIAN_POINT('Ctrl Pts',(38.2443930389404,263.915834356047,24.8538453138252)) ;
#101643=CARTESIAN_POINT('Ctrl Pts',(39.2354460092399,263.838513718924,23.3119105951427)) ;
#101644=CARTESIAN_POINT('Ctrl Pts',(41.0676934453923,263.761193081802,23.2607656185202)) ;
#101645=CARTESIAN_POINT('Ctrl Pts',(42.1432197226157,263.68387244468,24.745013193681)) ;
#101646=CARTESIAN_POINT('Ctrl Pts',(41.5240469724972,263.606551807558,26.4702322372449)) ;
#101647=CARTESIAN_POINT('Ctrl Pts',(39.7501671894346,263.529231170436,26.9318399560365)) ;
#101648=CARTESIAN_POINT('Ctrl Pts',(38.3685802199036,263.451910533313,25.7272777520254)) ;
#101649=CARTESIAN_POINT('Ctrl Pts',(38.5842101857908,263.374589896191,23.9070254611293)) ;
#101650=CARTESIAN_POINT('Ctrl Pts',(40.2089365236457,263.297269259069,23.0586014244381)) ;
#101651=CARTESIAN_POINT('Ctrl Pts',(41.8259723438625,263.219948621947,23.9217907880872)) ;
#101652=CARTESIAN_POINT('Ctrl Pts',(42.024768426902,263.142627984825,25.7440990447097)) ;
#101653=CARTESIAN_POINT('Ctrl Pts',(40.6326685573906,263.065307347703,26.9356693706473)) ;
#101654=CARTESIAN_POINT('Ctrl Pts',(38.8622468345652,262.98798671058,26.4588048179041)) ;
#101655=CARTESIAN_POINT('Ctrl Pts',(38.2609927628238,262.910666073458,24.7267081853047)) ;
#101656=CARTESIAN_POINT('Ctrl Pts',(38.984606102359,262.859118982043,23.7476731864398)) ;
#101657=CARTESIAN_POINT('Ctrl Pts',(39.4733401651905,262.833345436336,23.5123226518935)) ;
#101658=CARTESIAN_POINT('Ctrl Pts',(39.3461468006825,265.,23.2506310193419)) ;
#101659=CARTESIAN_POINT('Ctrl Pts',(39.2836598899885,265.,23.2857349597673)) ;
#101660=CARTESIAN_POINT('Ctrl Pts',(39.2234111410066,265.,23.3242492614719)) ;
#101661=CARTESIAN_POINT('Ctrl Pts',(39.1657274309582,265.,23.3661502764215)) ;
#101662=CARTESIAN_POINT('Ctrl Pts',(39.1551609910745,265.,23.3738256592144)) ;
#101663=CARTESIAN_POINT('Ctrl Pts',(39.1446806995909,265.,23.3816147975325)) ;
#101664=CARTESIAN_POINT('Ctrl Pts',(39.1342886811881,265.,23.3895176998347)) ;
#101665=CARTESIAN_POINT('Ctrl Pts',(39.0771212535977,265.,23.4329922759572)) ;
#101666=CARTESIAN_POINT('Ctrl Pts',(39.0226219173678,265.,23.4799068195409)) ;
#101667=CARTESIAN_POINT('Ctrl Pts',(38.9709292782328,265.,23.5299202960438)) ;
#101668=CARTESIAN_POINT('Ctrl Pts',(38.9227381202054,265.,23.576546032125)) ;
#101669=CARTESIAN_POINT('Ctrl Pts',(38.8769864064487,265.,23.6258661246551)) ;
#101670=CARTESIAN_POINT('Ctrl Pts',(38.833820414566,265.,23.677624408559)) ;
#101671=CARTESIAN_POINT('Ctrl Pts',(38.821574354322,265.,23.6923080758435)) ;
#101672=CARTESIAN_POINT('Ctrl Pts',(38.8095366203122,265.,23.7071880609811)) ;
#101673=CARTESIAN_POINT('Ctrl Pts',(38.7977110827752,265.,23.7222586759874)) ;
#101674=CARTESIAN_POINT('Ctrl Pts',(38.7880459026511,265.,23.7345761041094)) ;
#101675=CARTESIAN_POINT('Ctrl Pts',(38.7785200200342,265.,23.7470243724434)) ;
#101676=CARTESIAN_POINT('Ctrl Pts',(38.7691522808314,265.,23.7595775114929)) ;
#101677=CARTESIAN_POINT('Ctrl Pts',(38.7262247635429,265.,23.8171020733859)) ;
#101678=CARTESIAN_POINT('Ctrl Pts',(38.6865461566725,265.,23.8769100637447)) ;
#101679=CARTESIAN_POINT('Ctrl Pts',(38.6502422519169,265.,23.9386580305023)) ;
#101680=CARTESIAN_POINT('Ctrl Pts',(38.6140626397624,265.,24.000194592579)) ;
#101681=CARTESIAN_POINT('Ctrl Pts',(38.5812343178059,265.,24.0636589136051)) ;
#101682=CARTESIAN_POINT('Ctrl Pts',(38.5519287182427,265.,24.1287322580849)) ;
#101683=CARTESIAN_POINT('Ctrl Pts',(38.5217417171236,265.,24.1957627625593)) ;
#101684=CARTESIAN_POINT('Ctrl Pts',(38.4952918231741,265.,24.2645016083237)) ;
#101685=CARTESIAN_POINT('Ctrl Pts',(38.4728246435875,265.,24.3346069226516)) ;
#101686=CARTESIAN_POINT('Ctrl Pts',(38.468243329867,265.,24.3489021944358)) ;
#101687=CARTESIAN_POINT('Ctrl Pts',(38.4638278256027,265.,24.363254272894)) ;
#101688=CARTESIAN_POINT('Ctrl Pts',(38.4595805403143,265.,24.3776602266839)) ;
#101689=CARTESIAN_POINT('Ctrl Pts',(38.4560842396259,265.,24.3895189888661)) ;
#101690=CARTESIAN_POINT('Ctrl Pts',(38.4527017324949,265.,24.4014153269738)) ;
#101691=CARTESIAN_POINT('Ctrl Pts',(38.4494386829816,265.,24.4133310106522)) ;
#101692=CARTESIAN_POINT('Ctrl Pts',(38.4310468428157,265.,24.4804925259125)) ;
#101693=CARTESIAN_POINT('Ctrl Pts',(38.4164092350366,265.,24.54838861124)) ;
#101694=CARTESIAN_POINT('Ctrl Pts',(38.4056782411265,265.,24.6167188869397)) ;
#101695=CARTESIAN_POINT('Ctrl Pts',(38.3952678533935,265.,24.6830076827303)) ;
#101696=CARTESIAN_POINT('Ctrl Pts',(38.3885340905771,265.,24.7497059721214)) ;
#101697=CARTESIAN_POINT('Ctrl Pts',(38.3856640111701,265.,24.8165403736793)) ;
#101698=CARTESIAN_POINT('Ctrl Pts',(38.3832741020044,265.,24.872193241152)) ;
#101699=CARTESIAN_POINT('Ctrl Pts',(38.3835639723321,265.,24.927940723159)) ;
#101700=CARTESIAN_POINT('Ctrl Pts',(38.3866687294949,265.,24.9836192786205)) ;
#101701=CARTESIAN_POINT('Ctrl Pts',(38.3882598861759,265.,25.0121539758162)) ;
#101702=CARTESIAN_POINT('Ctrl Pts',(38.3905908183162,265.,25.0406704514666)) ;
#101703=CARTESIAN_POINT('Ctrl Pts',(38.3936513495387,265.,25.0691458950175)) ;
#101704=CARTESIAN_POINT('Ctrl Pts',(38.395335821027,265.,25.0848183614257)) ;
#101705=CARTESIAN_POINT('Ctrl Pts',(38.3972421531076,265.,25.1004833988623)) ;
#101706=CARTESIAN_POINT('Ctrl Pts',(38.3993642663105,265.,25.1161068307743)) ;
#101707=CARTESIAN_POINT('Ctrl Pts',(38.4084656882497,265.,25.1831133626456)) ;
#101708=CARTESIAN_POINT('Ctrl Pts',(38.421539478526,265.,25.2494500685674)) ;
#101709=CARTESIAN_POINT('Ctrl Pts',(38.4383668000559,265.,25.3148382144289)) ;
#101710=CARTESIAN_POINT('Ctrl Pts',(38.4553537568912,265.,25.3808466762818)) ;
#101711=CARTESIAN_POINT('Ctrl Pts',(38.4761663756549,265.,25.4458894365213)) ;
#101712=CARTESIAN_POINT('Ctrl Pts',(38.5006298528874,265.,25.5096610392952)) ;
#101713=CARTESIAN_POINT('Ctrl Pts',(38.5178779680934,265.,25.5546235743043)) ;
#101714=CARTESIAN_POINT('Ctrl Pts',(38.5369420027397,265.,25.598953840897)) ;
#101715=CARTESIAN_POINT('Ctrl Pts',(38.5577731540934,265.,25.6425354268357)) ;
#101716=CARTESIAN_POINT('Ctrl Pts',(38.5703022633925,265.,25.6687480179875)) ;
#101717=CARTESIAN_POINT('Ctrl Pts',(38.5834708216211,265.,25.6946896051629)) ;
#101718=CARTESIAN_POINT('Ctrl Pts',(38.597269718404,265.,25.7203330944085)) ;
#101719=CARTESIAN_POINT('Ctrl Pts',(38.6055041589436,265.,25.7356357516239)) ;
#101720=CARTESIAN_POINT('Ctrl Pts',(38.6139658244209,265.,25.7508366888722)) ;
#101721=CARTESIAN_POINT('Ctrl Pts',(38.6226370628273,265.,25.7659031711737)) ;
#101722=CARTESIAN_POINT('Ctrl Pts',(38.6561962222617,265.,25.8242130062832)) ;
#101723=CARTESIAN_POINT('Ctrl Pts',(38.6929261030111,265.,25.8805809342695)) ;
#101724=CARTESIAN_POINT('Ctrl Pts',(38.7326680429986,265.,25.9347034985894)) ;
#101725=CARTESIAN_POINT('Ctrl Pts',(38.7659314020797,265.,25.9800032069564)) ;
#101726=CARTESIAN_POINT('Ctrl Pts',(38.8013057749095,265.,26.0237296971601)) ;
#101727=CARTESIAN_POINT('Ctrl Pts',(38.8387166266962,265.,26.0656831084018)) ;
#101728=CARTESIAN_POINT('Ctrl Pts',(38.8518657159005,265.,26.0804288070559)) ;
#101729=CARTESIAN_POINT('Ctrl Pts',(38.8652665170064,265.,26.0949552572956)) ;
#101730=CARTESIAN_POINT('Ctrl Pts',(38.878916191547,265.,26.1092530611772)) ;
#101731=CARTESIAN_POINT('Ctrl Pts',(38.8880474805062,265.,26.1188179323643)) ;
#101732=CARTESIAN_POINT('Ctrl Pts',(38.8972834111552,265.,26.1282734040428)) ;
#101733=CARTESIAN_POINT('Ctrl Pts',(38.9066223963459,265.,26.137616745478)) ;
#101734=CARTESIAN_POINT('Ctrl Pts',(38.9528504522405,265.,26.1838663648201)) ;
#101735=CARTESIAN_POINT('Ctrl Pts',(39.0016043595963,265.,26.2273752673832)) ;
#101736=CARTESIAN_POINT('Ctrl Pts',(39.0527559256757,265.,26.2678349102572)) ;
#101737=CARTESIAN_POINT('Ctrl Pts',(39.1039074917551,265.,26.3082945531311)) ;
#101738=CARTESIAN_POINT('Ctrl Pts',(39.1574572962527,265.,26.3457057053902)) ;
#101739=CARTESIAN_POINT('Ctrl Pts',(39.2133011547203,265.,26.3797087969272)) ;
#101740=CARTESIAN_POINT('Ctrl Pts',(39.2174083575791,265.,26.3822096555462)) ;
#101741=CARTESIAN_POINT('Ctrl Pts',(39.2215279781247,265.,26.3846920529582)) ;
#101742=CARTESIAN_POINT('Ctrl Pts',(39.225659978706,265.,26.3871558334356)) ;
#101743=CARTESIAN_POINT('Origin',(40.2,265.,25.0213203435596)) ;
#101744=CARTESIAN_POINT('Origin',(40.2,255.,25.0213203435596)) ;
#117143=UNCERTAINTY_MEASURE_WITH_UNIT(LENGTH_MEASURE(0.01),#117171,
'DISTANCE_ACCURACY_VALUE',
'Maximum model space distance between geometric entities at asserted c
onnectivities') ;
#117147=UNCERTAINTY_MEASURE_WITH_UNIT(LENGTH_MEASURE(0.01),#117171,
'DISTANCE_ACCURACY_VALUE',
'Maximum model space distance between geometric entities at asserted c
onnectivities') ;
#117166=(
GEOMETRIC_REPRESENTATION_CONTEXT(3)
GLOBAL_UNCERTAINTY_ASSIGNED_CONTEXT((#117143))
GLOBAL_UNIT_ASSIGNED_CONTEXT((#117171,#117173,#117174))
REPRESENTATION_CONTEXT('','3D')
) ;
#117170=(
GEOMETRIC_REPRESENTATION_CONTEXT(3)
GLOBAL_UNCERTAINTY_ASSIGNED_CONTEXT((#117147))
GLOBAL_UNIT_ASSIGNED_CONTEXT((#117171,#117173,#117174))
REPRESENTATION_CONTEXT('','3D')
) ;
#117171=(
LENGTH_UNIT()
NAMED_UNIT(*)
SI_UNIT(.MILLI.,.METRE.)
) ;
#117173=(
NAMED_UNIT(*)
PLANE_ANGLE_UNIT()
SI_UNIT($,.RADIAN.)
) ;
#117174=(
NAMED_UNIT(*)
SI_UNIT($,.STERADIAN.)
SOLID_ANGLE_UNIT()
) ;
#117193=SHAPE_DEFINITION_REPRESENTATION(#117215,#117258) ;
#117215=PRODUCT_DEFINITION_SHAPE('',$,#117281) ;
#117258=SHAPE_REPRESENTATION('',(#54027),#117166) ;
#117262=PRODUCT_DEFINITION_CONTEXT('part definition',#117330,'design') ;
#117281=PRODUCT_DEFINITION('Knob_Shaft','Knob_Shaft',#117303,#117262) ;
#117303=PRODUCT_DEFINITION_FORMATION('',$,#117350) ;
#117330=APPLICATION_CONTEXT(
'Core Data for Automotive Mechanical Design Process') ;
#117331=PRODUCT_CONTEXT('part definition',#117330,'mechanical') ;
#117350=PRODUCT('Knob_Shaft','Knob_Shaft',$,(#117331)) ;
#117355=PRESENTATION_STYLE_ASSIGNMENT((#117357)) ;
#117357=SURFACE_STYLE_USAGE(.BOTH.,#117359) ;
#117359=SURFACE_SIDE_STYLE('',(#117361)) ;
#117361=SURFACE_STYLE_FILL_AREA(#117363) ;
#117363=FILL_AREA_STYLE('Opaque(160,160,160)',(#117365)) ;
#117365=FILL_AREA_STYLE_COLOUR('Opaque(160,160,160)',#117367) ;
#117367=COLOUR_RGB('Opaque(160,160,160)', 0.09019608, 0.27058824, 0.51372549) ;
ENDSEC;
END-ISO-10303-21;
